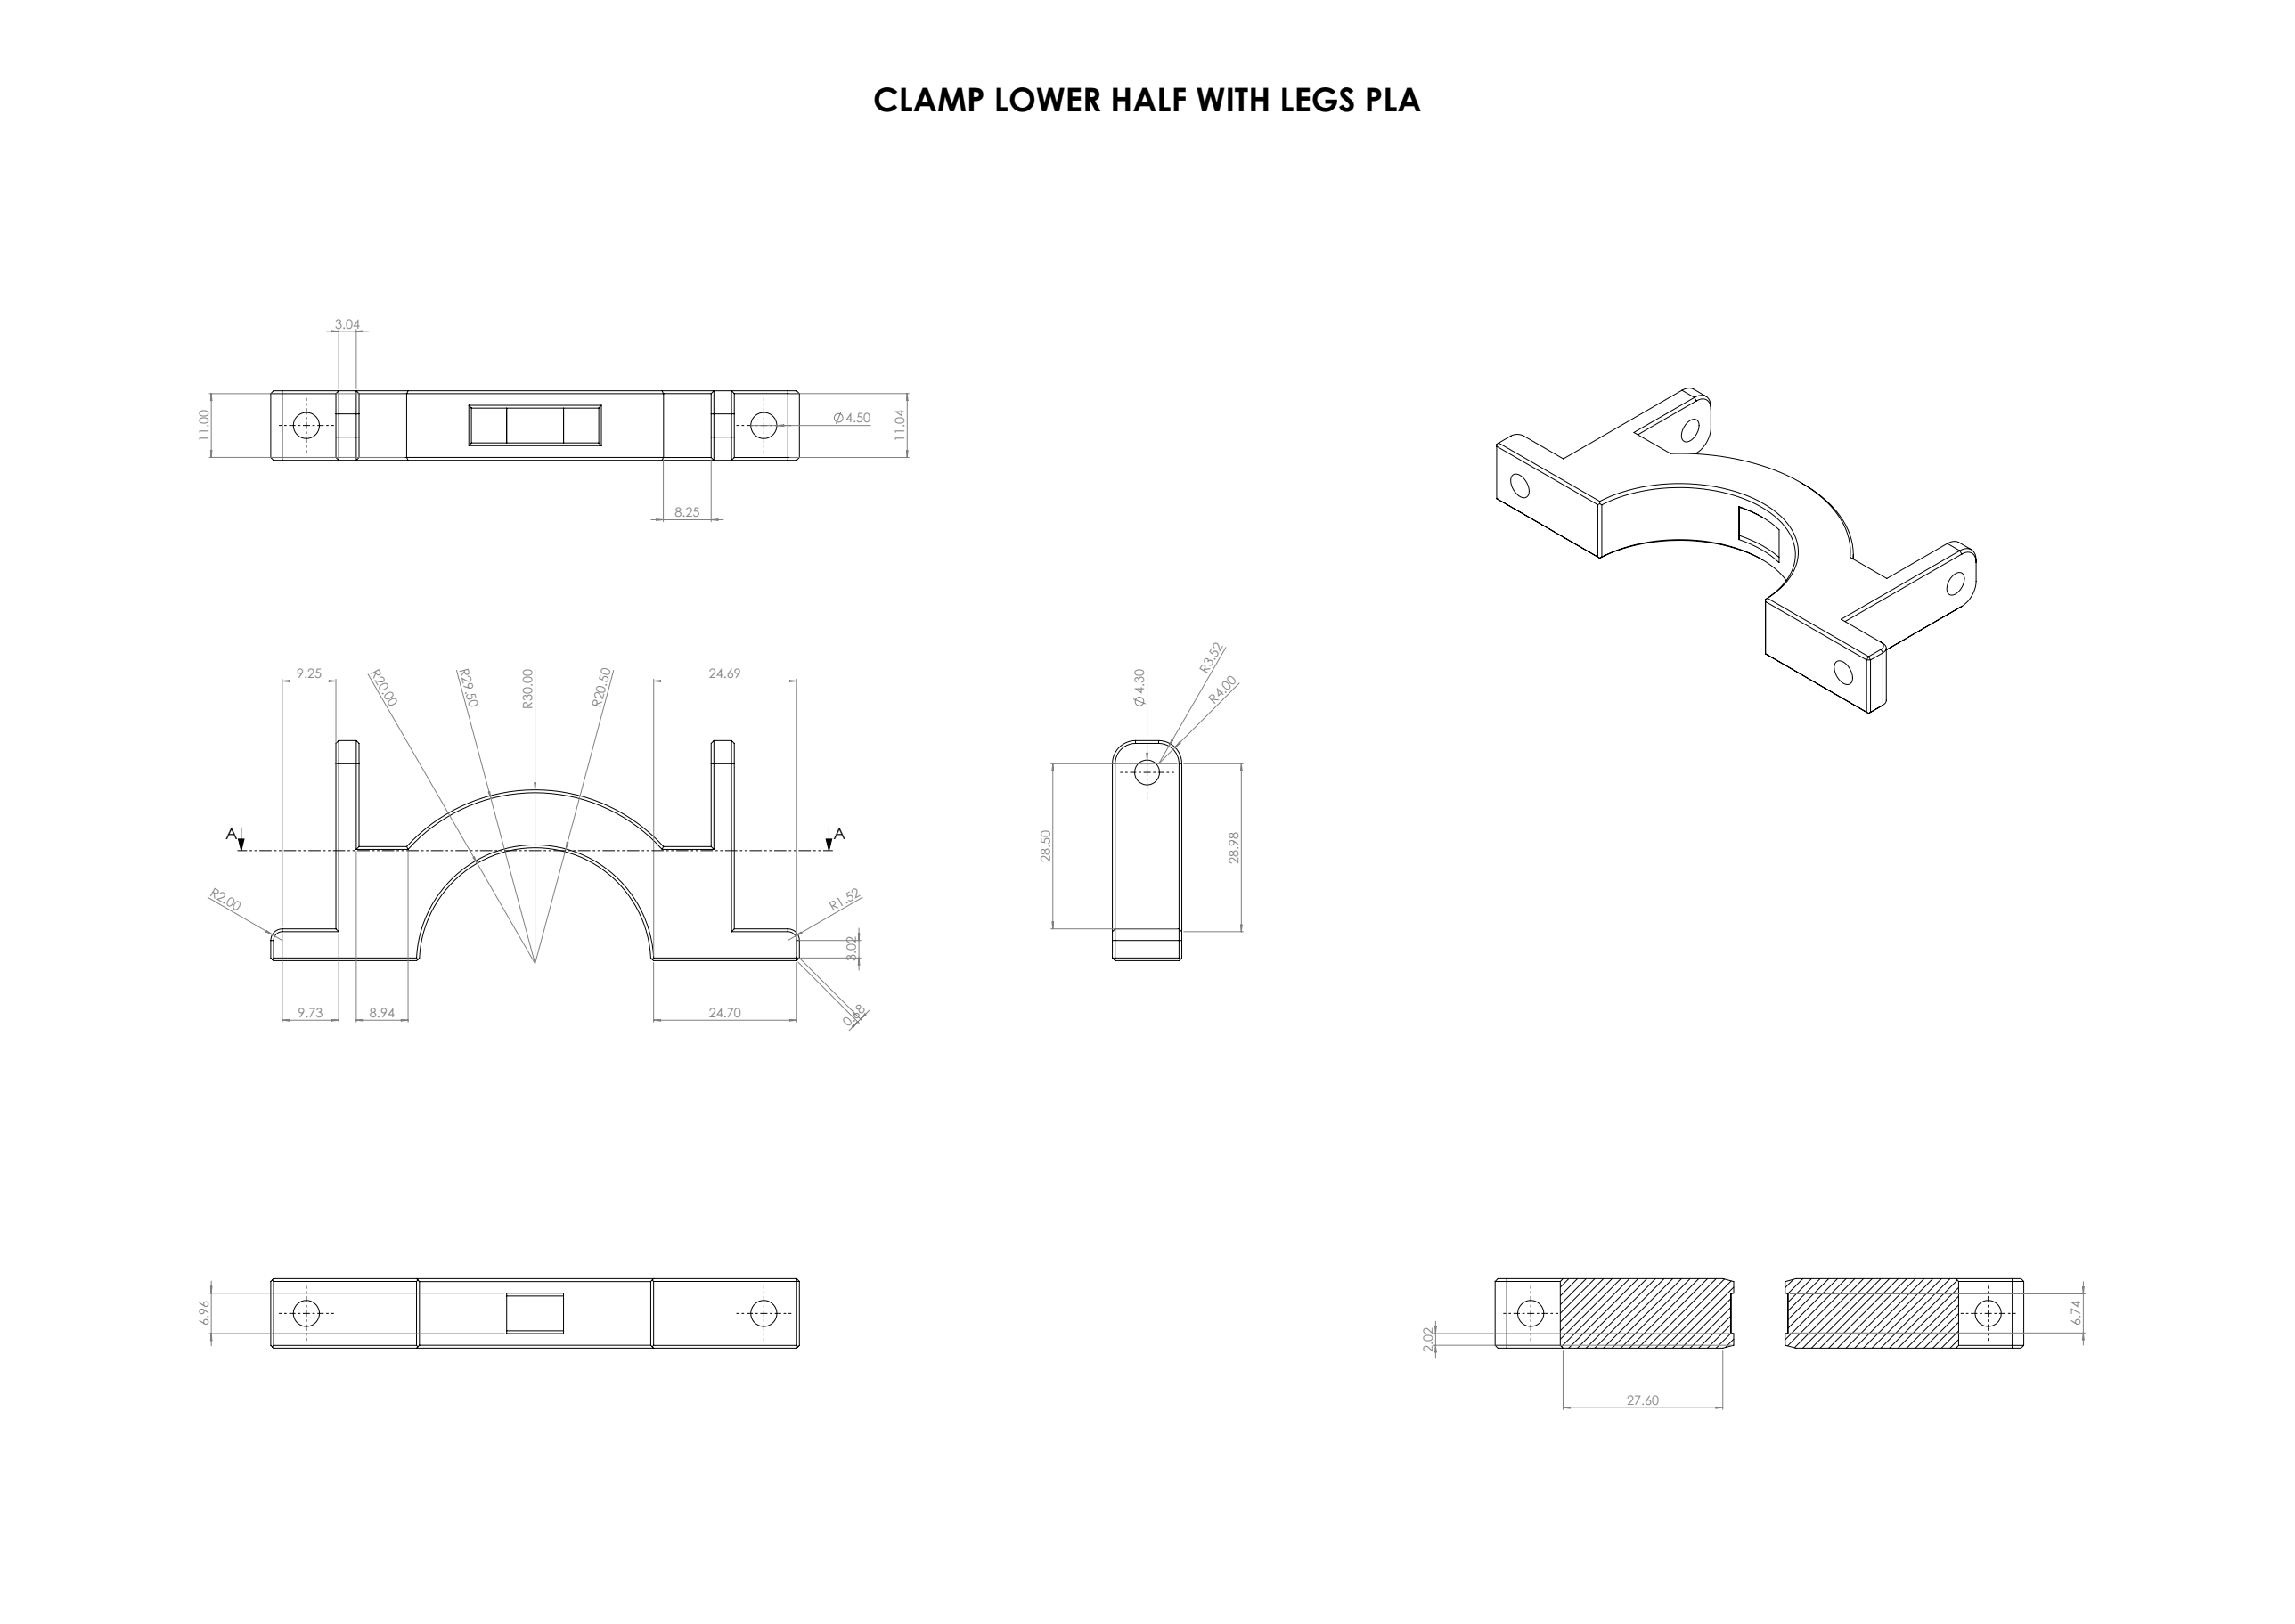
ISO-10303-21;
HEADER;
/* Generated by software containing ST-Developer
 * from STEP Tools, Inc. (www.steptools.com) 
 */

FILE_DESCRIPTION(
/* description */ (''),
/* implementation_level */ '2;1');

FILE_NAME(
/* name */ '02_Clamp_Lower_Half_with_Legs_PLA.step',
/* time_stamp */ '2026-10-21T02:01:14-07:00',
/* author */ (''),
/* organization */ (''),
/* preprocessor_version */ 'ST-DEVELOPER v20.2',
/* originating_system */ 'Autodesk Translation Framework v15.15.0.0',
/* authorisation */ '');

FILE_SCHEMA (('AUTOMOTIVE_DESIGN { 1 0 10303 214 3 1 1 }'));
ENDSEC;

DATA;
#10=MECHANICAL_DESIGN_GEOMETRIC_PRESENTATION_REPRESENTATION('',(#615),#37181);
#120=B_SPLINE_CURVE_WITH_KNOTS('',3,(#20379,#20380,#20381,#20382),
 .UNSPECIFIED.,.F.,.F.,(4,4),(-0.0159210516924088,0.),.UNSPECIFIED.);
#121=B_SPLINE_CURVE_WITH_KNOTS('',3,(#20385,#20386,#20387,#20388),
 .UNSPECIFIED.,.F.,.F.,(4,4),(-0.0159210527656447,0.),.UNSPECIFIED.);
#122=B_SPLINE_CURVE_WITH_KNOTS('',3,(#20391,#20392,#20393,#20394),
 .UNSPECIFIED.,.F.,.F.,(4,4),(-0.0159210517190927,0.),.UNSPECIFIED.);
#123=B_SPLINE_CURVE_WITH_KNOTS('',3,(#20397,#20398,#20399,#20400),
 .UNSPECIFIED.,.F.,.F.,(4,4),(-0.0159210527692958,0.),.UNSPECIFIED.);
#124=B_SPLINE_CURVE_WITH_KNOTS('',3,(#20440,#20441,#20442,#20443),
 .UNSPECIFIED.,.F.,.F.,(4,4),(-0.0698067370947057,0.),.UNSPECIFIED.);
#125=B_SPLINE_CURVE_WITH_KNOTS('',3,(#20446,#20447,#20448,#20449),
 .UNSPECIFIED.,.F.,.F.,(4,4),(-0.0698065886608642,0.),.UNSPECIFIED.);
#126=B_SPLINE_CURVE_WITH_KNOTS('',3,(#20455,#20456,#20457,#20458),
 .UNSPECIFIED.,.F.,.F.,(4,4),(-0.0698067370949415,0.),.UNSPECIFIED.);
#127=B_SPLINE_CURVE_WITH_KNOTS('',3,(#20461,#20462,#20463,#20464),
 .UNSPECIFIED.,.F.,.F.,(4,4),(-0.0698065886603473,0.),.UNSPECIFIED.);
#589=SHAPE_REPRESENTATION_RELATIONSHIP('SRR','None',#37239,#602);
#602=ADVANCED_BREP_SHAPE_REPRESENTATION('',(#628),#37169);
#615=STYLED_ITEM('',(#37387),#628);
#628=MANIFOLD_SOLID_BREP('Body1',#14777);
#644=FACE_BOUND('',#2261,.T.);
#645=FACE_BOUND('',#2293,.T.);
#646=FACE_BOUND('',#2303,.T.);
#647=FACE_BOUND('',#2305,.T.);
#648=FACE_BOUND('',#2313,.T.);
#649=FACE_BOUND('',#2321,.T.);
#650=FACE_BOUND('',#2336,.T.);
#651=FACE_BOUND('',#2339,.T.);
#652=FACE_BOUND('',#2351,.T.);
#653=FACE_BOUND('',#2354,.T.);
#696=CYLINDRICAL_SURFACE('',#15034,4.);
#697=CYLINDRICAL_SURFACE('',#15036,4.);
#698=CYLINDRICAL_SURFACE('',#15051,2.);
#699=CYLINDRICAL_SURFACE('',#15094,20.);
#700=CYLINDRICAL_SURFACE('',#15116,30.);
#701=CYLINDRICAL_SURFACE('',#15125,2.25);
#702=CYLINDRICAL_SURFACE('',#15126,2.25);
#703=CYLINDRICAL_SURFACE('',#15128,2.15);
#704=CYLINDRICAL_SURFACE('',#15130,2.15);
#705=CYLINDRICAL_SURFACE('',#15131,4.);
#706=CYLINDRICAL_SURFACE('',#15132,4.);
#707=CYLINDRICAL_SURFACE('',#15133,2.);
#971=CIRCLE('',#15000,4.);
#972=CIRCLE('',#15001,3.52);
#973=CIRCLE('',#15004,4.);
#974=CIRCLE('',#15005,3.52);
#975=CIRCLE('',#15009,2.15);
#976=CIRCLE('',#15015,2.);
#977=CIRCLE('',#15016,1.52);
#978=CIRCLE('',#15019,4.);
#979=CIRCLE('',#15020,3.52);
#980=CIRCLE('',#15023,4.);
#981=CIRCLE('',#15024,3.52);
#982=CIRCLE('',#15027,2.);
#983=CIRCLE('',#15028,1.52);
#984=CIRCLE('',#15031,29.5);
#985=CIRCLE('',#15032,1.52);
#986=CIRCLE('',#15033,20.5);
#987=CIRCLE('',#15038,20.5);
#988=CIRCLE('',#15039,1.52);
#989=CIRCLE('',#15040,29.5);
#990=CIRCLE('',#15048,2.);
#991=CIRCLE('',#15052,2.);
#992=CIRCLE('',#15057,2.25);
#993=CIRCLE('',#15063,4.);
#994=CIRCLE('',#15064,3.52);
#995=CIRCLE('',#15067,4.);
#996=CIRCLE('',#15068,3.52);
#997=CIRCLE('',#15071,2.25);
#998=CIRCLE('',#15073,2.15);
#999=CIRCLE('',#15077,4.);
#1000=CIRCLE('',#15078,3.52);
#1001=CIRCLE('',#15081,4.);
#1002=CIRCLE('',#15082,3.52);
#1003=CIRCLE('',#15085,2.15);
#1004=CIRCLE('',#15090,20.);
#1005=CIRCLE('',#15093,20.);
#1006=CIRCLE('',#15095,20.);
#1007=CIRCLE('',#15096,20.);
#1008=CIRCLE('',#15101,20.48);
#1009=CIRCLE('',#15103,20.48);
#1010=CIRCLE('',#15105,29.52);
#1011=CIRCLE('',#15110,30.);
#1012=CIRCLE('',#15112,30.);
#1013=CIRCLE('',#15113,29.52);
#1014=CIRCLE('',#15117,30.);
#1015=CIRCLE('',#15118,30.);
#1016=CIRCLE('',#15121,2.25);
#1017=CIRCLE('',#15127,2.25);
#1018=CIRCLE('',#15129,2.15);
#1291=CONICAL_SURFACE('',#14999,3.76,0.785398163397446);
#1292=CONICAL_SURFACE('',#15003,3.76,0.785398163397446);
#1293=CONICAL_SURFACE('',#15014,1.76,0.78539816339745);
#1294=CONICAL_SURFACE('',#15018,3.76,0.785398163397446);
#1295=CONICAL_SURFACE('',#15022,3.76,0.785398163397446);
#1296=CONICAL_SURFACE('',#15026,1.76,0.78539816339745);
#1297=CONICAL_SURFACE('',#15047,1.76,0.785398163397452);
#1298=CONICAL_SURFACE('',#15059,1.76,0.785398163397452);
#1299=CONICAL_SURFACE('',#15062,3.76,0.785398163397446);
#1300=CONICAL_SURFACE('',#15066,3.76,0.785398163397446);
#1301=CONICAL_SURFACE('',#15076,3.76,0.785398163397446);
#1302=CONICAL_SURFACE('',#15080,3.76,0.785398163397446);
#1303=CONICAL_SURFACE('',#15089,20.25,0.785398163397446);
#1304=CONICAL_SURFACE('',#15092,20.25,0.785398163397446);
#1305=CONICAL_SURFACE('',#15100,20.24,0.785398163397448);
#1306=CONICAL_SURFACE('',#15102,20.24,0.785398163397449);
#1307=CONICAL_SURFACE('',#15109,29.76,0.785398163397449);
#1308=CONICAL_SURFACE('',#15111,29.76,0.785398163397448);
#1309=CONICAL_SURFACE('',#15119,29.75,0.785398163397446);
#1310=CONICAL_SURFACE('',#15122,29.75,0.785398163397446);
#1410=FACE_OUTER_BOUND('',#2254,.T.);
#1411=FACE_OUTER_BOUND('',#2255,.T.);
#1412=FACE_OUTER_BOUND('',#2256,.T.);
#1413=FACE_OUTER_BOUND('',#2257,.T.);
#1414=FACE_OUTER_BOUND('',#2258,.T.);
#1415=FACE_OUTER_BOUND('',#2259,.T.);
#1416=FACE_OUTER_BOUND('',#2260,.T.);
#1417=FACE_OUTER_BOUND('',#2262,.T.);
#1418=FACE_OUTER_BOUND('',#2263,.T.);
#1419=FACE_OUTER_BOUND('',#2264,.T.);
#1420=FACE_OUTER_BOUND('',#2265,.T.);
#1421=FACE_OUTER_BOUND('',#2266,.T.);
#1422=FACE_OUTER_BOUND('',#2267,.T.);
#1423=FACE_OUTER_BOUND('',#2268,.T.);
#1424=FACE_OUTER_BOUND('',#2269,.T.);
#1425=FACE_OUTER_BOUND('',#2270,.T.);
#1426=FACE_OUTER_BOUND('',#2271,.T.);
#1427=FACE_OUTER_BOUND('',#2272,.T.);
#1428=FACE_OUTER_BOUND('',#2273,.T.);
#1429=FACE_OUTER_BOUND('',#2274,.T.);
#1430=FACE_OUTER_BOUND('',#2275,.T.);
#1431=FACE_OUTER_BOUND('',#2276,.T.);
#1432=FACE_OUTER_BOUND('',#2277,.T.);
#1433=FACE_OUTER_BOUND('',#2278,.T.);
#1434=FACE_OUTER_BOUND('',#2279,.T.);
#1435=FACE_OUTER_BOUND('',#2280,.T.);
#1436=FACE_OUTER_BOUND('',#2281,.T.);
#1437=FACE_OUTER_BOUND('',#2282,.T.);
#1438=FACE_OUTER_BOUND('',#2283,.T.);
#1439=FACE_OUTER_BOUND('',#2284,.T.);
#1440=FACE_OUTER_BOUND('',#2285,.T.);
#1441=FACE_OUTER_BOUND('',#2286,.T.);
#1442=FACE_OUTER_BOUND('',#2287,.T.);
#1443=FACE_OUTER_BOUND('',#2288,.T.);
#1444=FACE_OUTER_BOUND('',#2289,.T.);
#1445=FACE_OUTER_BOUND('',#2290,.T.);
#1446=FACE_OUTER_BOUND('',#2291,.T.);
#1447=FACE_OUTER_BOUND('',#2292,.T.);
#1448=FACE_OUTER_BOUND('',#2294,.T.);
#1449=FACE_OUTER_BOUND('',#2295,.T.);
#1450=FACE_OUTER_BOUND('',#2296,.T.);
#1451=FACE_OUTER_BOUND('',#2297,.T.);
#1452=FACE_OUTER_BOUND('',#2298,.T.);
#1453=FACE_OUTER_BOUND('',#2299,.T.);
#1454=FACE_OUTER_BOUND('',#2300,.T.);
#1455=FACE_OUTER_BOUND('',#2301,.T.);
#1456=FACE_OUTER_BOUND('',#2302,.T.);
#1457=FACE_OUTER_BOUND('',#2304,.T.);
#1458=FACE_OUTER_BOUND('',#2306,.T.);
#1459=FACE_OUTER_BOUND('',#2307,.T.);
#1460=FACE_OUTER_BOUND('',#2308,.T.);
#1461=FACE_OUTER_BOUND('',#2309,.T.);
#1462=FACE_OUTER_BOUND('',#2310,.T.);
#1463=FACE_OUTER_BOUND('',#2311,.T.);
#1464=FACE_OUTER_BOUND('',#2312,.T.);
#1465=FACE_OUTER_BOUND('',#2314,.T.);
#1466=FACE_OUTER_BOUND('',#2315,.T.);
#1467=FACE_OUTER_BOUND('',#2316,.T.);
#1468=FACE_OUTER_BOUND('',#2317,.T.);
#1469=FACE_OUTER_BOUND('',#2318,.T.);
#1470=FACE_OUTER_BOUND('',#2319,.T.);
#1471=FACE_OUTER_BOUND('',#2320,.T.);
#1472=FACE_OUTER_BOUND('',#2322,.T.);
#1473=FACE_OUTER_BOUND('',#2323,.T.);
#1474=FACE_OUTER_BOUND('',#2324,.T.);
#1475=FACE_OUTER_BOUND('',#2325,.T.);
#1476=FACE_OUTER_BOUND('',#2326,.T.);
#1477=FACE_OUTER_BOUND('',#2327,.T.);
#1478=FACE_OUTER_BOUND('',#2328,.T.);
#1479=FACE_OUTER_BOUND('',#2329,.T.);
#1480=FACE_OUTER_BOUND('',#2330,.T.);
#1481=FACE_OUTER_BOUND('',#2331,.T.);
#1482=FACE_OUTER_BOUND('',#2332,.T.);
#1483=FACE_OUTER_BOUND('',#2333,.T.);
#1484=FACE_OUTER_BOUND('',#2334,.T.);
#1485=FACE_OUTER_BOUND('',#2335,.T.);
#1486=FACE_OUTER_BOUND('',#2337,.T.);
#1487=FACE_OUTER_BOUND('',#2338,.T.);
#1488=FACE_OUTER_BOUND('',#2340,.T.);
#1489=FACE_OUTER_BOUND('',#2341,.T.);
#1490=FACE_OUTER_BOUND('',#2342,.T.);
#1491=FACE_OUTER_BOUND('',#2343,.T.);
#1492=FACE_OUTER_BOUND('',#2344,.T.);
#1493=FACE_OUTER_BOUND('',#2345,.T.);
#1494=FACE_OUTER_BOUND('',#2346,.T.);
#1495=FACE_OUTER_BOUND('',#2347,.T.);
#1496=FACE_OUTER_BOUND('',#2348,.T.);
#1497=FACE_OUTER_BOUND('',#2349,.T.);
#1498=FACE_OUTER_BOUND('',#2350,.T.);
#1499=FACE_OUTER_BOUND('',#2352,.T.);
#1500=FACE_OUTER_BOUND('',#2353,.T.);
#2254=EDGE_LOOP('',(#9371,#9372,#9373,#9374));
#2255=EDGE_LOOP('',(#9375,#9376,#9377,#9378));
#2256=EDGE_LOOP('',(#9379,#9380,#9381,#9382));
#2257=EDGE_LOOP('',(#9383,#9384,#9385,#9386));
#2258=EDGE_LOOP('',(#9387,#9388,#9389,#9390));
#2259=EDGE_LOOP('',(#9391,#9392,#9393,#9394));
#2260=EDGE_LOOP('',(#9395,#9396,#9397,#9398,#9399,#9400));
#2261=EDGE_LOOP('',(#9401));
#2262=EDGE_LOOP('',(#9402,#9403,#9404,#9405,#9406,#9407));
#2263=EDGE_LOOP('',(#9408,#9409,#9410,#9411));
#2264=EDGE_LOOP('',(#9412,#9413,#9414,#9415));
#2265=EDGE_LOOP('',(#9416,#9417,#9418,#9419));
#2266=EDGE_LOOP('',(#9420,#9421,#9422,#9423));
#2267=EDGE_LOOP('',(#9424,#9425,#9426,#9427,#9428));
#2268=EDGE_LOOP('',(#9429,#9430,#9431,#9432));
#2269=EDGE_LOOP('',(#9433,#9434,#9435,#9436));
#2270=EDGE_LOOP('',(#9437,#9438,#9439,#9440));
#2271=EDGE_LOOP('',(#9441,#9442,#9443,#9444));
#2272=EDGE_LOOP('',(#9445,#9446,#9447,#9448));
#2273=EDGE_LOOP('',(#9449,#9450,#9451,#9452,#9453));
#2274=EDGE_LOOP('',(#9454,#9455,#9456,#9457,#9458,#9459,#9460,#9461,#9462,
#9463,#9464,#9465,#9466,#9467,#9468,#9469,#9470,#9471));
#2275=EDGE_LOOP('',(#9472,#9473,#9474,#9475));
#2276=EDGE_LOOP('',(#9476,#9477,#9478,#9479));
#2277=EDGE_LOOP('',(#9480,#9481,#9482,#9483));
#2278=EDGE_LOOP('',(#9484,#9485,#9486,#9487,#9488,#9489,#9490,#9491,#9492,
#9493,#9494,#9495,#9496,#9497,#9498,#9499,#9500,#9501));
#2279=EDGE_LOOP('',(#9502,#9503,#9504,#9505,#9506,#9507));
#2280=EDGE_LOOP('',(#9508,#9509,#9510,#9511));
#2281=EDGE_LOOP('',(#9512,#9513,#9514,#9515,#9516,#9517));
#2282=EDGE_LOOP('',(#9518,#9519,#9520));
#2283=EDGE_LOOP('',(#9521,#9522,#9523,#9524,#9525));
#2284=EDGE_LOOP('',(#9526,#9527,#9528,#9529));
#2285=EDGE_LOOP('',(#9530,#9531,#9532,#9533));
#2286=EDGE_LOOP('',(#9534,#9535,#9536,#9537));
#2287=EDGE_LOOP('',(#9538,#9539,#9540,#9541,#9542));
#2288=EDGE_LOOP('',(#9543,#9544,#9545,#9546));
#2289=EDGE_LOOP('',(#9547,#9548,#9549,#9550));
#2290=EDGE_LOOP('',(#9551,#9552,#9553,#9554,#9555));
#2291=EDGE_LOOP('',(#9556,#9557,#9558,#9559,#9560,#9561));
#2292=EDGE_LOOP('',(#9562,#9563,#9564,#9565));
#2293=EDGE_LOOP('',(#9566));
#2294=EDGE_LOOP('',(#9567,#9568,#9569,#9570,#9571,#9572));
#2295=EDGE_LOOP('',(#9573,#9574,#9575,#9576));
#2296=EDGE_LOOP('',(#9577,#9578,#9579,#9580));
#2297=EDGE_LOOP('',(#9581,#9582,#9583,#9584));
#2298=EDGE_LOOP('',(#9585,#9586,#9587,#9588));
#2299=EDGE_LOOP('',(#9589,#9590,#9591,#9592));
#2300=EDGE_LOOP('',(#9593,#9594,#9595,#9596));
#2301=EDGE_LOOP('',(#9597,#9598,#9599,#9600));
#2302=EDGE_LOOP('',(#9601,#9602,#9603,#9604));
#2303=EDGE_LOOP('',(#9605));
#2304=EDGE_LOOP('',(#9606,#9607,#9608,#9609,#9610,#9611));
#2305=EDGE_LOOP('',(#9612));
#2306=EDGE_LOOP('',(#9613,#9614,#9615,#9616));
#2307=EDGE_LOOP('',(#9617,#9618,#9619,#9620));
#2308=EDGE_LOOP('',(#9621,#9622,#9623,#9624));
#2309=EDGE_LOOP('',(#9625,#9626,#9627,#9628));
#2310=EDGE_LOOP('',(#9629,#9630,#9631,#9632));
#2311=EDGE_LOOP('',(#9633,#9634,#9635,#9636));
#2312=EDGE_LOOP('',(#9637,#9638,#9639,#9640,#9641,#9642));
#2313=EDGE_LOOP('',(#9643));
#2314=EDGE_LOOP('',(#9644,#9645,#9646,#9647));
#2315=EDGE_LOOP('',(#9648,#9649,#9650,#9651,#9652,#9653));
#2316=EDGE_LOOP('',(#9654,#9655,#9656,#9657,#9658,#9659));
#2317=EDGE_LOOP('',(#9660,#9661,#9662,#9663,#9664,#9665));
#2318=EDGE_LOOP('',(#9666,#9667,#9668,#9669));
#2319=EDGE_LOOP('',(#9670,#9671,#9672,#9673,#9674,#9675));
#2320=EDGE_LOOP('',(#9676,#9677,#9678,#9679));
#2321=EDGE_LOOP('',(#9680,#9681,#9682,#9683));
#2322=EDGE_LOOP('',(#9684,#9685,#9686,#9687,#9688,#9689));
#2323=EDGE_LOOP('',(#9690,#9691,#9692,#9693));
#2324=EDGE_LOOP('',(#9694,#9695,#9696,#9697));
#2325=EDGE_LOOP('',(#9698,#9699,#9700,#9701,#9702,#9703));
#2326=EDGE_LOOP('',(#9704,#9705,#9706,#9707,#9708,#9709));
#2327=EDGE_LOOP('',(#9710,#9711,#9712,#9713,#9714,#9715));
#2328=EDGE_LOOP('',(#9716,#9717,#9718,#9719,#9720,#9721));
#2329=EDGE_LOOP('',(#9722,#9723,#9724,#9725));
#2330=EDGE_LOOP('',(#9726,#9727,#9728,#9729));
#2331=EDGE_LOOP('',(#9730,#9731,#9732,#9733,#9734,#9735));
#2332=EDGE_LOOP('',(#9736,#9737,#9738,#9739,#9740,#9741));
#2333=EDGE_LOOP('',(#9742,#9743,#9744,#9745,#9746,#9747));
#2334=EDGE_LOOP('',(#9748,#9749,#9750,#9751,#9752,#9753));
#2335=EDGE_LOOP('',(#9754,#9755,#9756,#9757));
#2336=EDGE_LOOP('',(#9758,#9759,#9760,#9761));
#2337=EDGE_LOOP('',(#9762,#9763,#9764,#9765,#9766,#9767));
#2338=EDGE_LOOP('',(#9768,#9769,#9770,#9771));
#2339=EDGE_LOOP('',(#9772));
#2340=EDGE_LOOP('',(#9773,#9774,#9775,#9776,#9777,#9778));
#2341=EDGE_LOOP('',(#9779,#9780,#9781,#9782,#9783,#9784));
#2342=EDGE_LOOP('',(#9785,#9786,#9787,#9788,#9789,#9790));
#2343=EDGE_LOOP('',(#9791,#9792,#9793,#9794));
#2344=EDGE_LOOP('',(#9795,#9796,#9797,#9798));
#2345=EDGE_LOOP('',(#9799,#9800,#9801,#9802));
#2346=EDGE_LOOP('',(#9803,#9804,#9805,#9806));
#2347=EDGE_LOOP('',(#9807,#9808,#9809,#9810));
#2348=EDGE_LOOP('',(#9811,#9812,#9813,#9814));
#2349=EDGE_LOOP('',(#9815,#9816,#9817,#9818));
#2350=EDGE_LOOP('',(#9819,#9820,#9821,#9822));
#2351=EDGE_LOOP('',(#9823));
#2352=EDGE_LOOP('',(#9824,#9825,#9826,#9827));
#2353=EDGE_LOOP('',(#9828,#9829,#9830,#9831,#9832,#9833));
#2354=EDGE_LOOP('',(#9834));
#3114=(
BOUNDED_CURVE()
B_SPLINE_CURVE(2,(#20022,#20023,#20024),.UNSPECIFIED.,.F.,.F.)
B_SPLINE_CURVE_WITH_KNOTS((3,3),(0.,0.0711434865298028),.UNSPECIFIED.)
CURVE()
GEOMETRIC_REPRESENTATION_ITEM()
RATIONAL_B_SPLINE_CURVE((1.,1.,1.))
REPRESENTATION_ITEM('')
);
#3115=(
BOUNDED_CURVE()
B_SPLINE_CURVE(2,(#20032,#20033,#20034),.UNSPECIFIED.,.F.,.F.)
B_SPLINE_CURVE_WITH_KNOTS((3,3),(0.0811630519003425,0.084492689542221),
 .UNSPECIFIED.)
CURVE()
GEOMETRIC_REPRESENTATION_ITEM()
RATIONAL_B_SPLINE_CURVE((1.0000049607761,1.00000258214363,1.))
REPRESENTATION_ITEM('')
);
#3116=(
BOUNDED_CURVE()
B_SPLINE_CURVE(2,(#20038,#20039,#20040),.UNSPECIFIED.,.F.,.F.)
B_SPLINE_CURVE_WITH_KNOTS((3,3),(0.,0.00332963764187841),.UNSPECIFIED.)
CURVE()
GEOMETRIC_REPRESENTATION_ITEM()
RATIONAL_B_SPLINE_CURVE((1.,1.00000258214363,1.0000049607761))
REPRESENTATION_ITEM('')
);
#3117=(
BOUNDED_CURVE()
B_SPLINE_CURVE(2,(#20175,#20176,#20177),.UNSPECIFIED.,.F.,.F.)
B_SPLINE_CURVE_WITH_KNOTS((3,3),(0.0429017134859085,0.0855944597309053),
 .UNSPECIFIED.)
CURVE()
GEOMETRIC_REPRESENTATION_ITEM()
RATIONAL_B_SPLINE_CURVE((1.,1.,1.))
REPRESENTATION_ITEM('')
);
#3118=(
BOUNDED_CURVE()
B_SPLINE_CURVE(2,(#20183,#20184,#20185),.UNSPECIFIED.,.F.,.F.)
B_SPLINE_CURVE_WITH_KNOTS((3,3),(0.,0.0711434865298028),.UNSPECIFIED.)
CURVE()
GEOMETRIC_REPRESENTATION_ITEM()
RATIONAL_B_SPLINE_CURVE((1.,1.,1.))
REPRESENTATION_ITEM('')
);
#3119=(
BOUNDED_CURVE()
B_SPLINE_CURVE(2,(#20192,#20193,#20194),.UNSPECIFIED.,.F.,.F.)
B_SPLINE_CURVE_WITH_KNOTS((3,3),(0.081163051900335,0.0844926895422209),
 .UNSPECIFIED.)
CURVE()
GEOMETRIC_REPRESENTATION_ITEM()
RATIONAL_B_SPLINE_CURVE((1.00000496077593,1.00000258214354,1.))
REPRESENTATION_ITEM('')
);
#3120=(
BOUNDED_CURVE()
B_SPLINE_CURVE(2,(#20197,#20198,#20199),.UNSPECIFIED.,.F.,.F.)
B_SPLINE_CURVE_WITH_KNOTS((3,3),(0.,0.00332963764188661),.UNSPECIFIED.)
CURVE()
GEOMETRIC_REPRESENTATION_ITEM()
RATIONAL_B_SPLINE_CURVE((1.,1.00000258214354,1.00000496077593))
REPRESENTATION_ITEM('')
);
#3121=(
BOUNDED_CURVE()
B_SPLINE_CURVE(2,(#20231,#20232,#20233),.UNSPECIFIED.,.F.,.F.)
B_SPLINE_CURVE_WITH_KNOTS((3,3),(0.,0.0426927462449967),.UNSPECIFIED.)
CURVE()
GEOMETRIC_REPRESENTATION_ITEM()
RATIONAL_B_SPLINE_CURVE((1.,1.,1.))
REPRESENTATION_ITEM('')
);
#3122=(
BOUNDED_CURVE()
B_SPLINE_CURVE(2,(#20250,#20251,#20252),.UNSPECIFIED.,.F.,.F.)
B_SPLINE_CURVE_WITH_KNOTS((3,3),(0.0429017134858602,0.0855944597309048),
 .UNSPECIFIED.)
CURVE()
GEOMETRIC_REPRESENTATION_ITEM()
RATIONAL_B_SPLINE_CURVE((1.,1.,1.))
REPRESENTATION_ITEM('')
);
#3123=(
BOUNDED_CURVE()
B_SPLINE_CURVE(2,(#20259,#20260,#20261),.UNSPECIFIED.,.F.,.F.)
B_SPLINE_CURVE_WITH_KNOTS((3,3),(0.043419103644769,0.0876516150043356),
 .UNSPECIFIED.)
CURVE()
GEOMETRIC_REPRESENTATION_ITEM()
RATIONAL_B_SPLINE_CURVE((1.00007900493187,1.00007974496581,1.))
REPRESENTATION_ITEM('')
);
#3124=(
BOUNDED_CURVE()
B_SPLINE_CURVE(2,(#20264,#20265,#20266),.UNSPECIFIED.,.F.,.F.)
B_SPLINE_CURVE_WITH_KNOTS((3,3),(0.,0.044232511359626),.UNSPECIFIED.)
CURVE()
GEOMETRIC_REPRESENTATION_ITEM()
RATIONAL_B_SPLINE_CURVE((1.,1.00007974496639,1.00007900493244))
REPRESENTATION_ITEM('')
);
#3125=(
BOUNDED_CURVE()
B_SPLINE_CURVE(2,(#20309,#20310,#20311),.UNSPECIFIED.,.F.,.F.)
B_SPLINE_CURVE_WITH_KNOTS((3,3),(0.,0.0711434865298029),.UNSPECIFIED.)
CURVE()
GEOMETRIC_REPRESENTATION_ITEM()
RATIONAL_B_SPLINE_CURVE((1.,1.,1.))
REPRESENTATION_ITEM('')
);
#3126=(
BOUNDED_CURVE()
B_SPLINE_CURVE(2,(#20335,#20336,#20337),.UNSPECIFIED.,.F.,.F.)
B_SPLINE_CURVE_WITH_KNOTS((3,3),(0.,0.0711434865298029),.UNSPECIFIED.)
CURVE()
GEOMETRIC_REPRESENTATION_ITEM()
RATIONAL_B_SPLINE_CURVE((1.,1.,1.))
REPRESENTATION_ITEM('')
);
#3127=(
BOUNDED_CURVE()
B_SPLINE_CURVE(2,(#20340,#20341,#20342),.UNSPECIFIED.,.F.,.F.)
B_SPLINE_CURVE_WITH_KNOTS((3,3),(0.,0.0426927462450447),.UNSPECIFIED.)
CURVE()
GEOMETRIC_REPRESENTATION_ITEM()
RATIONAL_B_SPLINE_CURVE((1.,1.,1.))
REPRESENTATION_ITEM('')
);
#3128=(
BOUNDED_CURVE()
B_SPLINE_CURVE(2,(#20354,#20355,#20356),.UNSPECIFIED.,.F.,.F.)
B_SPLINE_CURVE_WITH_KNOTS((3,3),(0.0434191036447888,0.0876516150043351),
 .UNSPECIFIED.)
CURVE()
GEOMETRIC_REPRESENTATION_ITEM()
RATIONAL_B_SPLINE_CURVE((1.00007900493244,1.00007974496639,1.))
REPRESENTATION_ITEM('')
);
#3129=(
BOUNDED_CURVE()
B_SPLINE_CURVE(2,(#20361,#20362,#20363),.UNSPECIFIED.,.F.,.F.)
B_SPLINE_CURVE_WITH_KNOTS((3,3),(0.,0.0442325113596284),.UNSPECIFIED.)
CURVE()
GEOMETRIC_REPRESENTATION_ITEM()
RATIONAL_B_SPLINE_CURVE((1.,1.00007974496678,1.00007900493282))
REPRESENTATION_ITEM('')
);
#3130=(
BOUNDED_CURVE()
B_SPLINE_CURVE(2,(#20405,#20406,#20407),.UNSPECIFIED.,.F.,.F.)
B_SPLINE_CURVE_WITH_KNOTS((3,3),(-3.26709460117384,-3.09375460254933),
 .UNSPECIFIED.)
CURVE()
GEOMETRIC_REPRESENTATION_ITEM()
RATIONAL_B_SPLINE_CURVE((1.22511255627814,1.2314549978879,1.23649074068738))
REPRESENTATION_ITEM('')
);
#3131=(
BOUNDED_CURVE()
B_SPLINE_CURVE(2,(#20408,#20409,#20410),.UNSPECIFIED.,.F.,.F.)
B_SPLINE_CURVE_WITH_KNOTS((3,3),(-1.75772269823236,-1.58438269960785),
 .UNSPECIFIED.)
CURVE()
GEOMETRIC_REPRESENTATION_ITEM()
RATIONAL_B_SPLINE_CURVE((1.23649074068738,1.2314549978879,1.22511255627814))
REPRESENTATION_ITEM('')
);
#3132=(
BOUNDED_CURVE()
B_SPLINE_CURVE(2,(#20413,#20414,#20415),.UNSPECIFIED.,.F.,.F.)
B_SPLINE_CURVE_WITH_KNOTS((3,3),(-1.75772269823236,-1.58438269960785),
 .UNSPECIFIED.)
CURVE()
GEOMETRIC_REPRESENTATION_ITEM()
RATIONAL_B_SPLINE_CURVE((1.23649074068738,1.2314549978879,1.22511255627814))
REPRESENTATION_ITEM('')
);
#3133=(
BOUNDED_CURVE()
B_SPLINE_CURVE(2,(#20418,#20419,#20420),.UNSPECIFIED.,.F.,.F.)
B_SPLINE_CURVE_WITH_KNOTS((3,3),(-3.26709460117384,-3.09375460254933),
 .UNSPECIFIED.)
CURVE()
GEOMETRIC_REPRESENTATION_ITEM()
RATIONAL_B_SPLINE_CURVE((1.22511255627814,1.2314549978879,1.23649074068738))
REPRESENTATION_ITEM('')
);
#3134=(
BOUNDED_CURVE()
B_SPLINE_CURVE(2,(#20466,#20467,#20468),.UNSPECIFIED.,.F.,.F.)
B_SPLINE_CURVE_WITH_KNOTS((3,3),(-0.360391606906832,-0.356059784727892),
 .UNSPECIFIED.)
CURVE()
GEOMETRIC_REPRESENTATION_ITEM()
RATIONAL_B_SPLINE_CURVE((1.0105812122411,1.01053365079744,1.01048570399065))
REPRESENTATION_ITEM('')
);
#3135=(
BOUNDED_CURVE()
B_SPLINE_CURVE(2,(#20470,#20471,#20472),.UNSPECIFIED.,.F.,.F.)
B_SPLINE_CURVE_WITH_KNOTS((3,3),(-1.43398872568548,-1.42965690350654),
 .UNSPECIFIED.)
CURVE()
GEOMETRIC_REPRESENTATION_ITEM()
RATIONAL_B_SPLINE_CURVE((1.01048570399065,1.01053365079744,1.0105812122411))
REPRESENTATION_ITEM('')
);
#3136=(
BOUNDED_CURVE()
B_SPLINE_CURVE(2,(#20476,#20477,#20478),.UNSPECIFIED.,.F.,.F.)
B_SPLINE_CURVE_WITH_KNOTS((3,3),(-1.43398872568546,-1.42965690350652),
 .UNSPECIFIED.)
CURVE()
GEOMETRIC_REPRESENTATION_ITEM()
RATIONAL_B_SPLINE_CURVE((1.01048570399063,1.01053365079743,1.01058121224108))
REPRESENTATION_ITEM('')
);
#3137=(
BOUNDED_CURVE()
B_SPLINE_CURVE(2,(#20481,#20482,#20483),.UNSPECIFIED.,.F.,.F.)
B_SPLINE_CURVE_WITH_KNOTS((3,3),(-0.360391606906842,-0.356059784727902),
 .UNSPECIFIED.)
CURVE()
GEOMETRIC_REPRESENTATION_ITEM()
RATIONAL_B_SPLINE_CURVE((1.01058121224108,1.01053365079743,1.01048570399063))
REPRESENTATION_ITEM('')
);
#3267=LINE('',#19988,#4506);
#3268=LINE('',#19990,#4507);
#3269=LINE('',#19992,#4508);
#3270=LINE('',#19993,#4509);
#3271=LINE('',#19998,#4510);
#3272=LINE('',#20003,#4511);
#3273=LINE('',#20004,#4512);
#3274=LINE('',#20005,#4513);
#3275=LINE('',#20010,#4514);
#3276=LINE('',#20014,#4515);
#3277=LINE('',#20016,#4516);
#3278=LINE('',#20017,#4517);
#3279=LINE('',#20020,#4518);
#3280=LINE('',#20025,#4519);
#3281=LINE('',#20027,#4520);
#3282=LINE('',#20036,#4521);
#3283=LINE('',#20041,#4522);
#3284=LINE('',#20045,#4523);
#3285=LINE('',#20047,#4524);
#3286=LINE('',#20049,#4525);
#3287=LINE('',#20050,#4526);
#3288=LINE('',#20054,#4527);
#3289=LINE('',#20056,#4528);
#3290=LINE('',#20058,#4529);
#3291=LINE('',#20059,#4530);
#3292=LINE('',#20062,#4531);
#3293=LINE('',#20064,#4532);
#3294=LINE('',#20065,#4533);
#3295=LINE('',#20069,#4534);
#3296=LINE('',#20075,#4535);
#3297=LINE('',#20076,#4536);
#3298=LINE('',#20078,#4537);
#3299=LINE('',#20079,#4538);
#3300=LINE('',#20083,#4539);
#3301=LINE('',#20089,#4540);
#3302=LINE('',#20090,#4541);
#3303=LINE('',#20091,#4542);
#3304=LINE('',#20095,#4543);
#3305=LINE('',#20099,#4544);
#3306=LINE('',#20100,#4545);
#3307=LINE('',#20105,#4546);
#3308=LINE('',#20110,#4547);
#3309=LINE('',#20111,#4548);
#3310=LINE('',#20113,#4549);
#3311=LINE('',#20114,#4550);
#3312=LINE('',#20117,#4551);
#3313=LINE('',#20121,#4552);
#3314=LINE('',#20123,#4553);
#3315=LINE('',#20125,#4554);
#3316=LINE('',#20127,#4555);
#3317=LINE('',#20129,#4556);
#3318=LINE('',#20133,#4557);
#3319=LINE('',#20135,#4558);
#3320=LINE('',#20138,#4559);
#3321=LINE('',#20139,#4560);
#3322=LINE('',#20141,#4561);
#3323=LINE('',#20143,#4562);
#3324=LINE('',#20145,#4563);
#3325=LINE('',#20148,#4564);
#3326=LINE('',#20152,#4565);
#3327=LINE('',#20154,#4566);
#3328=LINE('',#20158,#4567);
#3329=LINE('',#20160,#4568);
#3330=LINE('',#20162,#4569);
#3331=LINE('',#20164,#4570);
#3332=LINE('',#20166,#4571);
#3333=LINE('',#20170,#4572);
#3334=LINE('',#20172,#4573);
#3335=LINE('',#20174,#4574);
#3336=LINE('',#20180,#4575);
#3337=LINE('',#20182,#4576);
#3338=LINE('',#20188,#4577);
#3339=LINE('',#20190,#4578);
#3340=LINE('',#20196,#4579);
#3341=LINE('',#20202,#4580);
#3342=LINE('',#20204,#4581);
#3343=LINE('',#20205,#4582);
#3344=LINE('',#20209,#4583);
#3345=LINE('',#20210,#4584);
#3346=LINE('',#20212,#4585);
#3347=LINE('',#20213,#4586);
#3348=LINE('',#20216,#4587);
#3349=LINE('',#20217,#4588);
#3350=LINE('',#20221,#4589);
#3351=LINE('',#20224,#4590);
#3352=LINE('',#20225,#4591);
#3353=LINE('',#20229,#4592);
#3354=LINE('',#20230,#4593);
#3355=LINE('',#20236,#4594);
#3356=LINE('',#20239,#4595);
#3357=LINE('',#20241,#4596);
#3358=LINE('',#20243,#4597);
#3359=LINE('',#20244,#4598);
#3360=LINE('',#20247,#4599);
#3361=LINE('',#20249,#4600);
#3362=LINE('',#20254,#4601);
#3363=LINE('',#20263,#4602);
#3364=LINE('',#20268,#4603);
#3365=LINE('',#20271,#4604);
#3366=LINE('',#20272,#4605);
#3367=LINE('',#20275,#4606);
#3368=LINE('',#20276,#4607);
#3369=LINE('',#20280,#4608);
#3370=LINE('',#20285,#4609);
#3371=LINE('',#20287,#4610);
#3372=LINE('',#20288,#4611);
#3373=LINE('',#20291,#4612);
#3374=LINE('',#20295,#4613);
#3375=LINE('',#20297,#4614);
#3376=LINE('',#20305,#4615);
#3377=LINE('',#20306,#4616);
#3378=LINE('',#20307,#4617);
#3379=LINE('',#20315,#4618);
#3380=LINE('',#20321,#4619);
#3381=LINE('',#20322,#4620);
#3382=LINE('',#20323,#4621);
#3383=LINE('',#20326,#4622);
#3384=LINE('',#20330,#4623);
#3385=LINE('',#20344,#4624);
#3386=LINE('',#20346,#4625);
#3387=LINE('',#20347,#4626);
#3388=LINE('',#20349,#4627);
#3389=LINE('',#20350,#4628);
#3390=LINE('',#20358,#4629);
#3391=LINE('',#20366,#4630);
#3392=LINE('',#20369,#4631);
#3393=LINE('',#20373,#4632);
#3394=LINE('',#20376,#4633);
#3395=LINE('',#20384,#4634);
#3396=LINE('',#20396,#4635);
#3397=LINE('',#20423,#4636);
#3398=LINE('',#20425,#4637);
#3399=LINE('',#20429,#4638);
#3400=LINE('',#20430,#4639);
#3401=LINE('',#20433,#4640);
#3402=LINE('',#20434,#4641);
#3403=LINE('',#20438,#4642);
#3404=LINE('',#20445,#4643);
#3405=LINE('',#20453,#4644);
#3406=LINE('',#20460,#4645);
#3407=LINE('',#20486,#4646);
#3408=LINE('',#20487,#4647);
#3409=LINE('',#20488,#4648);
#3410=LINE('',#20499,#4649);
#3411=LINE('',#20502,#4650);
#3412=LINE('',#20505,#4651);
#3413=LINE('',#20510,#4652);
#3414=LINE('',#20512,#4653);
#3415=LINE('',#20514,#4654);
#3416=LINE('',#20516,#4655);
#3417=LINE('',#20518,#4656);
#3418=LINE('',#20520,#4657);
#4506=VECTOR('',#16321,10.);
#4507=VECTOR('',#16322,10.);
#4508=VECTOR('',#16323,10.);
#4509=VECTOR('',#16324,10.);
#4510=VECTOR('',#16329,10.);
#4511=VECTOR('',#16334,10.);
#4512=VECTOR('',#16335,10.);
#4513=VECTOR('',#16336,10.);
#4514=VECTOR('',#16341,10.);
#4515=VECTOR('',#16346,10.);
#4516=VECTOR('',#16347,10.);
#4517=VECTOR('',#16348,10.);
#4518=VECTOR('',#16351,10.);
#4519=VECTOR('',#16352,10.);
#4520=VECTOR('',#16355,10.);
#4521=VECTOR('',#16360,10.);
#4522=VECTOR('',#16361,10.);
#4523=VECTOR('',#16364,10.);
#4524=VECTOR('',#16365,10.);
#4525=VECTOR('',#16366,10.);
#4526=VECTOR('',#16367,10.);
#4527=VECTOR('',#16370,10.);
#4528=VECTOR('',#16371,10.);
#4529=VECTOR('',#16372,10.);
#4530=VECTOR('',#16373,10.);
#4531=VECTOR('',#16376,10.);
#4532=VECTOR('',#16377,10.);
#4533=VECTOR('',#16378,10.);
#4534=VECTOR('',#16381,10.);
#4535=VECTOR('',#16388,10.);
#4536=VECTOR('',#16389,10.);
#4537=VECTOR('',#16390,10.);
#4538=VECTOR('',#16391,10.);
#4539=VECTOR('',#16394,10.);
#4540=VECTOR('',#16401,10.);
#4541=VECTOR('',#16402,10.);
#4542=VECTOR('',#16403,10.);
#4543=VECTOR('',#16406,10.);
#4544=VECTOR('',#16413,10.);
#4545=VECTOR('',#16414,10.);
#4546=VECTOR('',#16419,10.);
#4547=VECTOR('',#16424,10.);
#4548=VECTOR('',#16425,10.);
#4549=VECTOR('',#16426,10.);
#4550=VECTOR('',#16427,10.);
#4551=VECTOR('',#16430,10.);
#4552=VECTOR('',#16433,10.);
#4553=VECTOR('',#16434,10.);
#4554=VECTOR('',#16435,10.);
#4555=VECTOR('',#16436,10.);
#4556=VECTOR('',#16437,10.);
#4557=VECTOR('',#16440,10.);
#4558=VECTOR('',#16441,10.);
#4559=VECTOR('',#16444,10.);
#4560=VECTOR('',#16445,10.);
#4561=VECTOR('',#16448,10.);
#4562=VECTOR('',#16451,10.);
#4563=VECTOR('',#16454,10.);
#4564=VECTOR('',#16457,10.);
#4565=VECTOR('',#16460,10.);
#4566=VECTOR('',#16461,10.);
#4567=VECTOR('',#16464,10.);
#4568=VECTOR('',#16465,10.);
#4569=VECTOR('',#16466,10.);
#4570=VECTOR('',#16467,10.);
#4571=VECTOR('',#16468,10.);
#4572=VECTOR('',#16473,10.);
#4573=VECTOR('',#16474,10.);
#4574=VECTOR('',#16475,10.);
#4575=VECTOR('',#16478,10.);
#4576=VECTOR('',#16479,10.);
#4577=VECTOR('',#16482,10.);
#4578=VECTOR('',#16483,10.);
#4579=VECTOR('',#16484,10.);
#4580=VECTOR('',#16487,10.);
#4581=VECTOR('',#16488,10.);
#4582=VECTOR('',#16489,10.);
#4583=VECTOR('',#16492,10.);
#4584=VECTOR('',#16493,10.);
#4585=VECTOR('',#16494,10.);
#4586=VECTOR('',#16495,10.);
#4587=VECTOR('',#16498,10.);
#4588=VECTOR('',#16499,10.);
#4589=VECTOR('',#16504,10.);
#4590=VECTOR('',#16507,10.);
#4591=VECTOR('',#16508,10.);
#4592=VECTOR('',#16511,10.);
#4593=VECTOR('',#16512,10.);
#4594=VECTOR('',#16515,10.);
#4595=VECTOR('',#16518,10.);
#4596=VECTOR('',#16521,10.);
#4597=VECTOR('',#16524,10.);
#4598=VECTOR('',#16525,10.);
#4599=VECTOR('',#16528,10.);
#4600=VECTOR('',#16529,10.);
#4601=VECTOR('',#16532,10.);
#4602=VECTOR('',#16537,10.);
#4603=VECTOR('',#16540,10.);
#4604=VECTOR('',#16543,10.);
#4605=VECTOR('',#16544,10.);
#4606=VECTOR('',#16547,10.);
#4607=VECTOR('',#16548,10.);
#4608=VECTOR('',#16551,10.);
#4609=VECTOR('',#16558,10.);
#4610=VECTOR('',#16559,10.);
#4611=VECTOR('',#16560,10.);
#4612=VECTOR('',#16563,10.);
#4613=VECTOR('',#16570,10.);
#4614=VECTOR('',#16573,10.);
#4615=VECTOR('',#16582,10.);
#4616=VECTOR('',#16583,10.);
#4617=VECTOR('',#16584,10.);
#4618=VECTOR('',#16589,10.);
#4619=VECTOR('',#16596,10.);
#4620=VECTOR('',#16597,10.);
#4621=VECTOR('',#16598,10.);
#4622=VECTOR('',#16601,10.);
#4623=VECTOR('',#16608,10.);
#4624=VECTOR('',#16617,10.);
#4625=VECTOR('',#16618,10.);
#4626=VECTOR('',#16619,10.);
#4627=VECTOR('',#16622,10.);
#4628=VECTOR('',#16623,10.);
#4629=VECTOR('',#16630,10.);
#4630=VECTOR('',#16637,10.);
#4631=VECTOR('',#16638,10.);
#4632=VECTOR('',#16641,10.);
#4633=VECTOR('',#16646,10.);
#4634=VECTOR('',#16649,10.);
#4635=VECTOR('',#16652,10.);
#4636=VECTOR('',#16663,10.);
#4637=VECTOR('',#16664,10.);
#4638=VECTOR('',#16667,10.);
#4639=VECTOR('',#16668,10.);
#4640=VECTOR('',#16671,10.);
#4641=VECTOR('',#16672,10.);
#4642=VECTOR('',#16675,10.);
#4643=VECTOR('',#16676,10.);
#4644=VECTOR('',#16679,10.);
#4645=VECTOR('',#16680,10.);
#4646=VECTOR('',#16693,10.);
#4647=VECTOR('',#16694,10.);
#4648=VECTOR('',#16695,10.);
#4649=VECTOR('',#16714,10.);
#4650=VECTOR('',#16719,2.25);
#4651=VECTOR('',#16722,2.25);
#4652=VECTOR('',#16729,2.15);
#4653=VECTOR('',#16732,2.15);
#4654=VECTOR('',#16735,10.);
#4655=VECTOR('',#16738,10.);
#4656=VECTOR('',#16741,10.);
#4657=VECTOR('',#16744,10.);
#5741=VERTEX_POINT('',#19986);
#5742=VERTEX_POINT('',#19987);
#5743=VERTEX_POINT('',#19989);
#5744=VERTEX_POINT('',#19991);
#5745=VERTEX_POINT('',#19995);
#5746=VERTEX_POINT('',#19997);
#5747=VERTEX_POINT('',#20001);
#5748=VERTEX_POINT('',#20002);
#5749=VERTEX_POINT('',#20007);
#5750=VERTEX_POINT('',#20009);
#5751=VERTEX_POINT('',#20013);
#5752=VERTEX_POINT('',#20015);
#5753=VERTEX_POINT('',#20019);
#5754=VERTEX_POINT('',#20021);
#5755=VERTEX_POINT('',#20028);
#5756=VERTEX_POINT('',#20031);
#5757=VERTEX_POINT('',#20035);
#5758=VERTEX_POINT('',#20037);
#5759=VERTEX_POINT('',#20043);
#5760=VERTEX_POINT('',#20044);
#5761=VERTEX_POINT('',#20046);
#5762=VERTEX_POINT('',#20048);
#5763=VERTEX_POINT('',#20052);
#5764=VERTEX_POINT('',#20053);
#5765=VERTEX_POINT('',#20055);
#5766=VERTEX_POINT('',#20057);
#5767=VERTEX_POINT('',#20061);
#5768=VERTEX_POINT('',#20063);
#5769=VERTEX_POINT('',#20067);
#5770=VERTEX_POINT('',#20068);
#5771=VERTEX_POINT('',#20073);
#5772=VERTEX_POINT('',#20074);
#5773=VERTEX_POINT('',#20077);
#5774=VERTEX_POINT('',#20081);
#5775=VERTEX_POINT('',#20082);
#5776=VERTEX_POINT('',#20087);
#5777=VERTEX_POINT('',#20088);
#5778=VERTEX_POINT('',#20093);
#5779=VERTEX_POINT('',#20094);
#5780=VERTEX_POINT('',#20102);
#5781=VERTEX_POINT('',#20104);
#5782=VERTEX_POINT('',#20108);
#5783=VERTEX_POINT('',#20109);
#5784=VERTEX_POINT('',#20112);
#5785=VERTEX_POINT('',#20116);
#5786=VERTEX_POINT('',#20118);
#5787=VERTEX_POINT('',#20120);
#5788=VERTEX_POINT('',#20122);
#5789=VERTEX_POINT('',#20124);
#5790=VERTEX_POINT('',#20126);
#5791=VERTEX_POINT('',#20128);
#5792=VERTEX_POINT('',#20130);
#5793=VERTEX_POINT('',#20132);
#5794=VERTEX_POINT('',#20134);
#5795=VERTEX_POINT('',#20136);
#5796=VERTEX_POINT('',#20147);
#5797=VERTEX_POINT('',#20149);
#5798=VERTEX_POINT('',#20151);
#5799=VERTEX_POINT('',#20153);
#5800=VERTEX_POINT('',#20155);
#5801=VERTEX_POINT('',#20157);
#5802=VERTEX_POINT('',#20159);
#5803=VERTEX_POINT('',#20161);
#5804=VERTEX_POINT('',#20163);
#5805=VERTEX_POINT('',#20165);
#5806=VERTEX_POINT('',#20169);
#5807=VERTEX_POINT('',#20171);
#5808=VERTEX_POINT('',#20173);
#5809=VERTEX_POINT('',#20179);
#5810=VERTEX_POINT('',#20181);
#5811=VERTEX_POINT('',#20187);
#5812=VERTEX_POINT('',#20189);
#5813=VERTEX_POINT('',#20191);
#5814=VERTEX_POINT('',#20195);
#5815=VERTEX_POINT('',#20201);
#5816=VERTEX_POINT('',#20203);
#5817=VERTEX_POINT('',#20207);
#5818=VERTEX_POINT('',#20208);
#5819=VERTEX_POINT('',#20211);
#5820=VERTEX_POINT('',#20215);
#5821=VERTEX_POINT('',#20219);
#5822=VERTEX_POINT('',#20223);
#5823=VERTEX_POINT('',#20227);
#5824=VERTEX_POINT('',#20228);
#5825=VERTEX_POINT('',#20235);
#5826=VERTEX_POINT('',#20237);
#5827=VERTEX_POINT('',#20246);
#5828=VERTEX_POINT('',#20248);
#5829=VERTEX_POINT('',#20255);
#5830=VERTEX_POINT('',#20258);
#5831=VERTEX_POINT('',#20262);
#5832=VERTEX_POINT('',#20270);
#5833=VERTEX_POINT('',#20274);
#5834=VERTEX_POINT('',#20278);
#5835=VERTEX_POINT('',#20279);
#5836=VERTEX_POINT('',#20284);
#5837=VERTEX_POINT('',#20286);
#5838=VERTEX_POINT('',#20290);
#5839=VERTEX_POINT('',#20298);
#5840=VERTEX_POINT('',#20301);
#5841=VERTEX_POINT('',#20304);
#5842=VERTEX_POINT('',#20313);
#5843=VERTEX_POINT('',#20314);
#5844=VERTEX_POINT('',#20319);
#5845=VERTEX_POINT('',#20320);
#5846=VERTEX_POINT('',#20325);
#5847=VERTEX_POINT('',#20332);
#5848=VERTEX_POINT('',#20339);
#5849=VERTEX_POINT('',#20343);
#5850=VERTEX_POINT('',#20345);
#5851=VERTEX_POINT('',#20352);
#5852=VERTEX_POINT('',#20360);
#5853=VERTEX_POINT('',#20367);
#5854=VERTEX_POINT('',#20368);
#5855=VERTEX_POINT('',#20370);
#5856=VERTEX_POINT('',#20372);
#5857=VERTEX_POINT('',#20378);
#5858=VERTEX_POINT('',#20383);
#5859=VERTEX_POINT('',#20390);
#5860=VERTEX_POINT('',#20395);
#5861=VERTEX_POINT('',#20402);
#5862=VERTEX_POINT('',#20403);
#5863=VERTEX_POINT('',#20412);
#5864=VERTEX_POINT('',#20416);
#5865=VERTEX_POINT('',#20422);
#5866=VERTEX_POINT('',#20424);
#5867=VERTEX_POINT('',#20426);
#5868=VERTEX_POINT('',#20428);
#5869=VERTEX_POINT('',#20432);
#5870=VERTEX_POINT('',#20436);
#5871=VERTEX_POINT('',#20437);
#5872=VERTEX_POINT('',#20439);
#5873=VERTEX_POINT('',#20444);
#5874=VERTEX_POINT('',#20451);
#5875=VERTEX_POINT('',#20452);
#5876=VERTEX_POINT('',#20454);
#5877=VERTEX_POINT('',#20459);
#5878=VERTEX_POINT('',#20475);
#5879=VERTEX_POINT('',#20479);
#5880=VERTEX_POINT('',#20485);
#5881=VERTEX_POINT('',#20495);
#5882=VERTEX_POINT('',#20504);
#5883=VERTEX_POINT('',#20508);
#7127=EDGE_CURVE('',#5741,#5742,#3267,.F.);
#7128=EDGE_CURVE('',#5742,#5743,#3268,.T.);
#7129=EDGE_CURVE('',#5743,#5744,#3269,.T.);
#7130=EDGE_CURVE('',#5744,#5741,#3270,.T.);
#7131=EDGE_CURVE('',#5743,#5745,#971,.T.);
#7132=EDGE_CURVE('',#5745,#5746,#3271,.T.);
#7133=EDGE_CURVE('',#5746,#5744,#972,.T.);
#7134=EDGE_CURVE('',#5747,#5748,#3272,.T.);
#7135=EDGE_CURVE('',#5748,#5746,#3273,.T.);
#7136=EDGE_CURVE('',#5745,#5747,#3274,.T.);
#7137=EDGE_CURVE('',#5747,#5749,#973,.T.);
#7138=EDGE_CURVE('',#5749,#5750,#3275,.T.);
#7139=EDGE_CURVE('',#5750,#5748,#974,.T.);
#7140=EDGE_CURVE('',#5751,#5750,#3276,.T.);
#7141=EDGE_CURVE('',#5749,#5752,#3277,.T.);
#7142=EDGE_CURVE('',#5752,#5751,#3278,.T.);
#7143=EDGE_CURVE('',#5752,#5753,#3279,.T.);
#7144=EDGE_CURVE('',#5753,#5754,#3114,.F.);
#7145=EDGE_CURVE('',#5754,#5751,#3280,.T.);
#7146=EDGE_CURVE('',#5741,#5751,#3281,.T.);
#7147=EDGE_CURVE('',#5755,#5755,#975,.T.);
#7148=EDGE_CURVE('',#5756,#5754,#3115,.F.);
#7149=EDGE_CURVE('',#5757,#5756,#3282,.T.);
#7150=EDGE_CURVE('',#5758,#5757,#3116,.F.);
#7151=EDGE_CURVE('',#5741,#5758,#3283,.T.);
#7152=EDGE_CURVE('',#5759,#5760,#3284,.T.);
#7153=EDGE_CURVE('',#5760,#5761,#3285,.T.);
#7154=EDGE_CURVE('',#5761,#5762,#3286,.T.);
#7155=EDGE_CURVE('',#5762,#5759,#3287,.T.);
#7156=EDGE_CURVE('',#5763,#5764,#3288,.T.);
#7157=EDGE_CURVE('',#5764,#5765,#3289,.T.);
#7158=EDGE_CURVE('',#5765,#5766,#3290,.T.);
#7159=EDGE_CURVE('',#5766,#5763,#3291,.T.);
#7160=EDGE_CURVE('',#5766,#5767,#3292,.T.);
#7161=EDGE_CURVE('',#5767,#5768,#3293,.T.);
#7162=EDGE_CURVE('',#5768,#5763,#3294,.T.);
#7163=EDGE_CURVE('',#5769,#5770,#3295,.T.);
#7164=EDGE_CURVE('',#5770,#5768,#976,.T.);
#7165=EDGE_CURVE('',#5767,#5769,#977,.T.);
#7166=EDGE_CURVE('',#5771,#5772,#3296,.T.);
#7167=EDGE_CURVE('',#5772,#5770,#3297,.T.);
#7168=EDGE_CURVE('',#5769,#5773,#3298,.T.);
#7169=EDGE_CURVE('',#5773,#5771,#3299,.T.);
#7170=EDGE_CURVE('',#5774,#5775,#3300,.T.);
#7171=EDGE_CURVE('',#5775,#5765,#978,.T.);
#7172=EDGE_CURVE('',#5764,#5774,#979,.T.);
#7173=EDGE_CURVE('',#5776,#5777,#3301,.T.);
#7174=EDGE_CURVE('',#5777,#5775,#3302,.T.);
#7175=EDGE_CURVE('',#5774,#5776,#3303,.T.);
#7176=EDGE_CURVE('',#5778,#5779,#3304,.T.);
#7177=EDGE_CURVE('',#5779,#5777,#980,.T.);
#7178=EDGE_CURVE('',#5776,#5778,#981,.T.);
#7179=EDGE_CURVE('',#5762,#5779,#3305,.T.);
#7180=EDGE_CURVE('',#5778,#5759,#3306,.T.);
#7181=EDGE_CURVE('',#5760,#5780,#982,.T.);
#7182=EDGE_CURVE('',#5780,#5781,#3307,.T.);
#7183=EDGE_CURVE('',#5781,#5761,#983,.T.);
#7184=EDGE_CURVE('',#5782,#5783,#3308,.T.);
#7185=EDGE_CURVE('',#5783,#5781,#3309,.T.);
#7186=EDGE_CURVE('',#5780,#5784,#3310,.T.);
#7187=EDGE_CURVE('',#5784,#5782,#3311,.T.);
#7188=EDGE_CURVE('',#5785,#5742,#3312,.T.);
#7189=EDGE_CURVE('',#5786,#5785,#984,.T.);
#7190=EDGE_CURVE('',#5787,#5786,#3313,.T.);
#7191=EDGE_CURVE('',#5788,#5787,#3314,.T.);
#7192=EDGE_CURVE('',#5789,#5788,#3315,.T.);
#7193=EDGE_CURVE('',#5790,#5789,#3316,.T.);
#7194=EDGE_CURVE('',#5791,#5790,#3317,.T.);
#7195=EDGE_CURVE('',#5792,#5791,#985,.T.);
#7196=EDGE_CURVE('',#5793,#5792,#3318,.T.);
#7197=EDGE_CURVE('',#5794,#5793,#3319,.T.);
#7198=EDGE_CURVE('',#5795,#5794,#986,.T.);
#7199=EDGE_CURVE('',#5773,#5795,#3320,.T.);
#7200=EDGE_CURVE('',#5743,#5765,#3321,.T.);
#7201=EDGE_CURVE('',#5775,#5745,#3322,.T.);
#7202=EDGE_CURVE('',#5747,#5777,#3323,.T.);
#7203=EDGE_CURVE('',#5779,#5749,#3324,.T.);
#7204=EDGE_CURVE('',#5796,#5783,#3325,.T.);
#7205=EDGE_CURVE('',#5797,#5796,#987,.T.);
#7206=EDGE_CURVE('',#5798,#5797,#3326,.T.);
#7207=EDGE_CURVE('',#5799,#5798,#3327,.T.);
#7208=EDGE_CURVE('',#5800,#5799,#988,.T.);
#7209=EDGE_CURVE('',#5801,#5800,#3328,.T.);
#7210=EDGE_CURVE('',#5802,#5801,#3329,.T.);
#7211=EDGE_CURVE('',#5803,#5802,#3330,.T.);
#7212=EDGE_CURVE('',#5804,#5803,#3331,.T.);
#7213=EDGE_CURVE('',#5805,#5804,#3332,.T.);
#7214=EDGE_CURVE('',#5753,#5805,#989,.T.);
#7215=EDGE_CURVE('',#5806,#5782,#3333,.T.);
#7216=EDGE_CURVE('',#5806,#5807,#3334,.T.);
#7217=EDGE_CURVE('',#5807,#5808,#3335,.T.);
#7218=EDGE_CURVE('',#5808,#5796,#3117,.T.);
#7219=EDGE_CURVE('',#5804,#5809,#3336,.F.);
#7220=EDGE_CURVE('',#5809,#5810,#3337,.T.);
#7221=EDGE_CURVE('',#5810,#5805,#3118,.F.);
#7222=EDGE_CURVE('',#5811,#5809,#3338,.T.);
#7223=EDGE_CURVE('',#5812,#5811,#3339,.T.);
#7224=EDGE_CURVE('',#5813,#5812,#3119,.F.);
#7225=EDGE_CURVE('',#5813,#5814,#3340,.T.);
#7226=EDGE_CURVE('',#5810,#5814,#3120,.F.);
#7227=EDGE_CURVE('',#5815,#5798,#3341,.T.);
#7228=EDGE_CURVE('',#5816,#5815,#3342,.T.);
#7229=EDGE_CURVE('',#5798,#5816,#3343,.T.);
#7230=EDGE_CURVE('',#5817,#5818,#3344,.T.);
#7231=EDGE_CURVE('',#5818,#5816,#3345,.T.);
#7232=EDGE_CURVE('',#5815,#5819,#3346,.T.);
#7233=EDGE_CURVE('',#5819,#5817,#3347,.T.);
#7234=EDGE_CURVE('',#5820,#5799,#3348,.T.);
#7235=EDGE_CURVE('',#5816,#5820,#3349,.T.);
#7236=EDGE_CURVE('',#5820,#5821,#990,.T.);
#7237=EDGE_CURVE('',#5821,#5800,#3350,.T.);
#7238=EDGE_CURVE('',#5822,#5801,#3351,.F.);
#7239=EDGE_CURVE('',#5821,#5822,#3352,.T.);
#7240=EDGE_CURVE('',#5823,#5824,#3353,.T.);
#7241=EDGE_CURVE('',#5824,#5815,#3354,.T.);
#7242=EDGE_CURVE('',#5797,#5823,#3121,.T.);
#7243=EDGE_CURVE('',#5820,#5825,#3355,.T.);
#7244=EDGE_CURVE('',#5826,#5825,#991,.T.);
#7245=EDGE_CURVE('',#5826,#5821,#3356,.T.);
#7246=EDGE_CURVE('',#5825,#5818,#3357,.T.);
#7247=EDGE_CURVE('',#5793,#5817,#3358,.T.);
#7248=EDGE_CURVE('',#5792,#5825,#3359,.T.);
#7249=EDGE_CURVE('',#5819,#5827,#3360,.T.);
#7250=EDGE_CURVE('',#5827,#5828,#3361,.T.);
#7251=EDGE_CURVE('',#5828,#5794,#3122,.T.);
#7252=EDGE_CURVE('',#5827,#5824,#3362,.T.);
#7253=EDGE_CURVE('',#5829,#5829,#992,.T.);
#7254=EDGE_CURVE('',#5823,#5830,#3123,.T.);
#7255=EDGE_CURVE('',#5830,#5831,#3363,.T.);
#7256=EDGE_CURVE('',#5831,#5828,#3124,.T.);
#7257=EDGE_CURVE('',#5791,#5826,#3364,.T.);
#7258=EDGE_CURVE('',#5832,#5826,#3365,.T.);
#7259=EDGE_CURVE('',#5790,#5832,#3366,.T.);
#7260=EDGE_CURVE('',#5822,#5833,#3367,.T.);
#7261=EDGE_CURVE('',#5833,#5802,#3368,.T.);
#7262=EDGE_CURVE('',#5834,#5835,#3369,.T.);
#7263=EDGE_CURVE('',#5835,#5802,#993,.T.);
#7264=EDGE_CURVE('',#5833,#5834,#994,.T.);
#7265=EDGE_CURVE('',#5834,#5836,#3370,.T.);
#7266=EDGE_CURVE('',#5836,#5837,#3371,.T.);
#7267=EDGE_CURVE('',#5837,#5835,#3372,.T.);
#7268=EDGE_CURVE('',#5838,#5789,#3373,.T.);
#7269=EDGE_CURVE('',#5789,#5837,#995,.T.);
#7270=EDGE_CURVE('',#5836,#5838,#996,.T.);
#7271=EDGE_CURVE('',#5838,#5832,#3374,.T.);
#7272=EDGE_CURVE('',#5832,#5822,#3375,.T.);
#7273=EDGE_CURVE('',#5839,#5839,#997,.T.);
#7274=EDGE_CURVE('',#5840,#5840,#998,.T.);
#7275=EDGE_CURVE('',#5811,#5841,#3376,.T.);
#7276=EDGE_CURVE('',#5841,#5788,#3377,.T.);
#7277=EDGE_CURVE('',#5787,#5811,#3378,.T.);
#7278=EDGE_CURVE('',#5786,#5812,#3125,.F.);
#7279=EDGE_CURVE('',#5842,#5843,#3379,.T.);
#7280=EDGE_CURVE('',#5843,#5788,#999,.T.);
#7281=EDGE_CURVE('',#5841,#5842,#1000,.T.);
#7282=EDGE_CURVE('',#5844,#5845,#3380,.T.);
#7283=EDGE_CURVE('',#5845,#5843,#3381,.T.);
#7284=EDGE_CURVE('',#5842,#5844,#3382,.T.);
#7285=EDGE_CURVE('',#5846,#5803,#3383,.T.);
#7286=EDGE_CURVE('',#5803,#5845,#1001,.T.);
#7287=EDGE_CURVE('',#5844,#5846,#1002,.T.);
#7288=EDGE_CURVE('',#5846,#5809,#3384,.T.);
#7289=EDGE_CURVE('',#5847,#5847,#1003,.T.);
#7290=EDGE_CURVE('',#5758,#5785,#3126,.F.);
#7291=EDGE_CURVE('',#5795,#5848,#3127,.T.);
#7292=EDGE_CURVE('',#5848,#5849,#3385,.T.);
#7293=EDGE_CURVE('',#5849,#5850,#3386,.T.);
#7294=EDGE_CURVE('',#5850,#5771,#3387,.T.);
#7295=EDGE_CURVE('',#5850,#5806,#3388,.T.);
#7296=EDGE_CURVE('',#5784,#5772,#3389,.T.);
#7297=EDGE_CURVE('',#5831,#5851,#1004,.T.);
#7298=EDGE_CURVE('',#5848,#5851,#3128,.T.);
#7299=EDGE_CURVE('',#5770,#5780,#3390,.T.);
#7300=EDGE_CURVE('',#5852,#5808,#3129,.T.);
#7301=EDGE_CURVE('',#5852,#5830,#1005,.T.);
#7302=EDGE_CURVE('',#5851,#5852,#3391,.T.);
#7303=EDGE_CURVE('',#5853,#5854,#3392,.T.);
#7304=EDGE_CURVE('',#5855,#5853,#1006,.T.);
#7305=EDGE_CURVE('',#5856,#5855,#3393,.T.);
#7306=EDGE_CURVE('',#5854,#5856,#1007,.T.);
#7307=EDGE_CURVE('',#5807,#5849,#3394,.T.);
#7308=EDGE_CURVE('',#5855,#5857,#120,.T.);
#7309=EDGE_CURVE('',#5857,#5858,#3395,.T.);
#7310=EDGE_CURVE('',#5858,#5856,#121,.T.);
#7311=EDGE_CURVE('',#5854,#5859,#122,.T.);
#7312=EDGE_CURVE('',#5859,#5860,#3396,.T.);
#7313=EDGE_CURVE('',#5860,#5853,#123,.T.);
#7314=EDGE_CURVE('',#5861,#5862,#1008,.T.);
#7315=EDGE_CURVE('',#5862,#5859,#3130,.T.);
#7316=EDGE_CURVE('',#5858,#5861,#3131,.T.);
#7317=EDGE_CURVE('',#5860,#5863,#3132,.T.);
#7318=EDGE_CURVE('',#5863,#5864,#1009,.T.);
#7319=EDGE_CURVE('',#5864,#5857,#3133,.T.);
#7320=EDGE_CURVE('',#5865,#5863,#3397,.T.);
#7321=EDGE_CURVE('',#5866,#5865,#3398,.T.);
#7322=EDGE_CURVE('',#5867,#5866,#1010,.T.);
#7323=EDGE_CURVE('',#5868,#5867,#3399,.T.);
#7324=EDGE_CURVE('',#5864,#5868,#3400,.T.);
#7325=EDGE_CURVE('',#5862,#5869,#3401,.T.);
#7326=EDGE_CURVE('',#5865,#5869,#3402,.T.);
#7327=EDGE_CURVE('',#5870,#5871,#3403,.T.);
#7328=EDGE_CURVE('',#5871,#5872,#124,.T.);
#7329=EDGE_CURVE('',#5872,#5873,#3404,.T.);
#7330=EDGE_CURVE('',#5873,#5870,#125,.T.);
#7331=EDGE_CURVE('',#5874,#5875,#3405,.T.);
#7332=EDGE_CURVE('',#5875,#5876,#126,.T.);
#7333=EDGE_CURVE('',#5876,#5877,#3406,.T.);
#7334=EDGE_CURVE('',#5877,#5874,#127,.T.);
#7335=EDGE_CURVE('',#5866,#5876,#3134,.T.);
#7336=EDGE_CURVE('',#5875,#5870,#1011,.T.);
#7337=EDGE_CURVE('',#5873,#5867,#3135,.T.);
#7338=EDGE_CURVE('',#5871,#5874,#1012,.T.);
#7339=EDGE_CURVE('',#5877,#5878,#3136,.T.);
#7340=EDGE_CURVE('',#5878,#5879,#1013,.T.);
#7341=EDGE_CURVE('',#5879,#5872,#3137,.T.);
#7342=EDGE_CURVE('',#5880,#5861,#3407,.T.);
#7343=EDGE_CURVE('',#5879,#5880,#3408,.T.);
#7344=EDGE_CURVE('',#5869,#5878,#3409,.T.);
#7345=EDGE_CURVE('',#5814,#5756,#1014,.T.);
#7346=EDGE_CURVE('',#5757,#5813,#1015,.T.);
#7347=EDGE_CURVE('',#5881,#5881,#1016,.T.);
#7348=EDGE_CURVE('',#5868,#5880,#3410,.T.);
#7349=EDGE_CURVE('',#5829,#5839,#3411,.T.);
#7350=EDGE_CURVE('',#5881,#5882,#3412,.T.);
#7351=EDGE_CURVE('',#5882,#5882,#1017,.T.);
#7352=EDGE_CURVE('',#5883,#5883,#1018,.T.);
#7353=EDGE_CURVE('',#5883,#5755,#3413,.T.);
#7354=EDGE_CURVE('',#5840,#5847,#3414,.T.);
#7355=EDGE_CURVE('',#5843,#5837,#3415,.T.);
#7356=EDGE_CURVE('',#5835,#5845,#3416,.T.);
#7357=EDGE_CURVE('',#5760,#5768,#3417,.T.);
#7358=EDGE_CURVE('',#5763,#5759,#3418,.T.);
#9371=ORIENTED_EDGE('',*,*,#7127,.T.);
#9372=ORIENTED_EDGE('',*,*,#7128,.T.);
#9373=ORIENTED_EDGE('',*,*,#7129,.T.);
#9374=ORIENTED_EDGE('',*,*,#7130,.T.);
#9375=ORIENTED_EDGE('',*,*,#7129,.F.);
#9376=ORIENTED_EDGE('',*,*,#7131,.T.);
#9377=ORIENTED_EDGE('',*,*,#7132,.T.);
#9378=ORIENTED_EDGE('',*,*,#7133,.T.);
#9379=ORIENTED_EDGE('',*,*,#7134,.T.);
#9380=ORIENTED_EDGE('',*,*,#7135,.T.);
#9381=ORIENTED_EDGE('',*,*,#7132,.F.);
#9382=ORIENTED_EDGE('',*,*,#7136,.T.);
#9383=ORIENTED_EDGE('',*,*,#7134,.F.);
#9384=ORIENTED_EDGE('',*,*,#7137,.T.);
#9385=ORIENTED_EDGE('',*,*,#7138,.T.);
#9386=ORIENTED_EDGE('',*,*,#7139,.T.);
#9387=ORIENTED_EDGE('',*,*,#7140,.T.);
#9388=ORIENTED_EDGE('',*,*,#7138,.F.);
#9389=ORIENTED_EDGE('',*,*,#7141,.T.);
#9390=ORIENTED_EDGE('',*,*,#7142,.T.);
#9391=ORIENTED_EDGE('',*,*,#7143,.T.);
#9392=ORIENTED_EDGE('',*,*,#7144,.T.);
#9393=ORIENTED_EDGE('',*,*,#7145,.T.);
#9394=ORIENTED_EDGE('',*,*,#7142,.F.);
#9395=ORIENTED_EDGE('',*,*,#7130,.F.);
#9396=ORIENTED_EDGE('',*,*,#7133,.F.);
#9397=ORIENTED_EDGE('',*,*,#7135,.F.);
#9398=ORIENTED_EDGE('',*,*,#7139,.F.);
#9399=ORIENTED_EDGE('',*,*,#7140,.F.);
#9400=ORIENTED_EDGE('',*,*,#7146,.F.);
#9401=ORIENTED_EDGE('',*,*,#7147,.T.);
#9402=ORIENTED_EDGE('',*,*,#7145,.F.);
#9403=ORIENTED_EDGE('',*,*,#7148,.F.);
#9404=ORIENTED_EDGE('',*,*,#7149,.F.);
#9405=ORIENTED_EDGE('',*,*,#7150,.F.);
#9406=ORIENTED_EDGE('',*,*,#7151,.F.);
#9407=ORIENTED_EDGE('',*,*,#7146,.T.);
#9408=ORIENTED_EDGE('',*,*,#7152,.T.);
#9409=ORIENTED_EDGE('',*,*,#7153,.T.);
#9410=ORIENTED_EDGE('',*,*,#7154,.T.);
#9411=ORIENTED_EDGE('',*,*,#7155,.T.);
#9412=ORIENTED_EDGE('',*,*,#7156,.T.);
#9413=ORIENTED_EDGE('',*,*,#7157,.T.);
#9414=ORIENTED_EDGE('',*,*,#7158,.T.);
#9415=ORIENTED_EDGE('',*,*,#7159,.T.);
#9416=ORIENTED_EDGE('',*,*,#7160,.T.);
#9417=ORIENTED_EDGE('',*,*,#7161,.T.);
#9418=ORIENTED_EDGE('',*,*,#7162,.T.);
#9419=ORIENTED_EDGE('',*,*,#7159,.F.);
#9420=ORIENTED_EDGE('',*,*,#7163,.T.);
#9421=ORIENTED_EDGE('',*,*,#7164,.T.);
#9422=ORIENTED_EDGE('',*,*,#7161,.F.);
#9423=ORIENTED_EDGE('',*,*,#7165,.T.);
#9424=ORIENTED_EDGE('',*,*,#7166,.T.);
#9425=ORIENTED_EDGE('',*,*,#7167,.T.);
#9426=ORIENTED_EDGE('',*,*,#7163,.F.);
#9427=ORIENTED_EDGE('',*,*,#7168,.T.);
#9428=ORIENTED_EDGE('',*,*,#7169,.T.);
#9429=ORIENTED_EDGE('',*,*,#7170,.T.);
#9430=ORIENTED_EDGE('',*,*,#7171,.T.);
#9431=ORIENTED_EDGE('',*,*,#7157,.F.);
#9432=ORIENTED_EDGE('',*,*,#7172,.T.);
#9433=ORIENTED_EDGE('',*,*,#7173,.T.);
#9434=ORIENTED_EDGE('',*,*,#7174,.T.);
#9435=ORIENTED_EDGE('',*,*,#7170,.F.);
#9436=ORIENTED_EDGE('',*,*,#7175,.T.);
#9437=ORIENTED_EDGE('',*,*,#7176,.T.);
#9438=ORIENTED_EDGE('',*,*,#7177,.T.);
#9439=ORIENTED_EDGE('',*,*,#7173,.F.);
#9440=ORIENTED_EDGE('',*,*,#7178,.T.);
#9441=ORIENTED_EDGE('',*,*,#7179,.T.);
#9442=ORIENTED_EDGE('',*,*,#7176,.F.);
#9443=ORIENTED_EDGE('',*,*,#7180,.T.);
#9444=ORIENTED_EDGE('',*,*,#7155,.F.);
#9445=ORIENTED_EDGE('',*,*,#7153,.F.);
#9446=ORIENTED_EDGE('',*,*,#7181,.T.);
#9447=ORIENTED_EDGE('',*,*,#7182,.T.);
#9448=ORIENTED_EDGE('',*,*,#7183,.T.);
#9449=ORIENTED_EDGE('',*,*,#7184,.T.);
#9450=ORIENTED_EDGE('',*,*,#7185,.T.);
#9451=ORIENTED_EDGE('',*,*,#7182,.F.);
#9452=ORIENTED_EDGE('',*,*,#7186,.T.);
#9453=ORIENTED_EDGE('',*,*,#7187,.T.);
#9454=ORIENTED_EDGE('',*,*,#7188,.F.);
#9455=ORIENTED_EDGE('',*,*,#7189,.F.);
#9456=ORIENTED_EDGE('',*,*,#7190,.F.);
#9457=ORIENTED_EDGE('',*,*,#7191,.F.);
#9458=ORIENTED_EDGE('',*,*,#7192,.F.);
#9459=ORIENTED_EDGE('',*,*,#7193,.F.);
#9460=ORIENTED_EDGE('',*,*,#7194,.F.);
#9461=ORIENTED_EDGE('',*,*,#7195,.F.);
#9462=ORIENTED_EDGE('',*,*,#7196,.F.);
#9463=ORIENTED_EDGE('',*,*,#7197,.F.);
#9464=ORIENTED_EDGE('',*,*,#7198,.F.);
#9465=ORIENTED_EDGE('',*,*,#7199,.F.);
#9466=ORIENTED_EDGE('',*,*,#7168,.F.);
#9467=ORIENTED_EDGE('',*,*,#7165,.F.);
#9468=ORIENTED_EDGE('',*,*,#7160,.F.);
#9469=ORIENTED_EDGE('',*,*,#7158,.F.);
#9470=ORIENTED_EDGE('',*,*,#7200,.F.);
#9471=ORIENTED_EDGE('',*,*,#7128,.F.);
#9472=ORIENTED_EDGE('',*,*,#7131,.F.);
#9473=ORIENTED_EDGE('',*,*,#7200,.T.);
#9474=ORIENTED_EDGE('',*,*,#7171,.F.);
#9475=ORIENTED_EDGE('',*,*,#7201,.T.);
#9476=ORIENTED_EDGE('',*,*,#7136,.F.);
#9477=ORIENTED_EDGE('',*,*,#7201,.F.);
#9478=ORIENTED_EDGE('',*,*,#7174,.F.);
#9479=ORIENTED_EDGE('',*,*,#7202,.F.);
#9480=ORIENTED_EDGE('',*,*,#7137,.F.);
#9481=ORIENTED_EDGE('',*,*,#7202,.T.);
#9482=ORIENTED_EDGE('',*,*,#7177,.F.);
#9483=ORIENTED_EDGE('',*,*,#7203,.T.);
#9484=ORIENTED_EDGE('',*,*,#7141,.F.);
#9485=ORIENTED_EDGE('',*,*,#7203,.F.);
#9486=ORIENTED_EDGE('',*,*,#7179,.F.);
#9487=ORIENTED_EDGE('',*,*,#7154,.F.);
#9488=ORIENTED_EDGE('',*,*,#7183,.F.);
#9489=ORIENTED_EDGE('',*,*,#7185,.F.);
#9490=ORIENTED_EDGE('',*,*,#7204,.F.);
#9491=ORIENTED_EDGE('',*,*,#7205,.F.);
#9492=ORIENTED_EDGE('',*,*,#7206,.F.);
#9493=ORIENTED_EDGE('',*,*,#7207,.F.);
#9494=ORIENTED_EDGE('',*,*,#7208,.F.);
#9495=ORIENTED_EDGE('',*,*,#7209,.F.);
#9496=ORIENTED_EDGE('',*,*,#7210,.F.);
#9497=ORIENTED_EDGE('',*,*,#7211,.F.);
#9498=ORIENTED_EDGE('',*,*,#7212,.F.);
#9499=ORIENTED_EDGE('',*,*,#7213,.F.);
#9500=ORIENTED_EDGE('',*,*,#7214,.F.);
#9501=ORIENTED_EDGE('',*,*,#7143,.F.);
#9502=ORIENTED_EDGE('',*,*,#7184,.F.);
#9503=ORIENTED_EDGE('',*,*,#7215,.F.);
#9504=ORIENTED_EDGE('',*,*,#7216,.T.);
#9505=ORIENTED_EDGE('',*,*,#7217,.T.);
#9506=ORIENTED_EDGE('',*,*,#7218,.T.);
#9507=ORIENTED_EDGE('',*,*,#7204,.T.);
#9508=ORIENTED_EDGE('',*,*,#7219,.T.);
#9509=ORIENTED_EDGE('',*,*,#7220,.T.);
#9510=ORIENTED_EDGE('',*,*,#7221,.T.);
#9511=ORIENTED_EDGE('',*,*,#7213,.T.);
#9512=ORIENTED_EDGE('',*,*,#7220,.F.);
#9513=ORIENTED_EDGE('',*,*,#7222,.F.);
#9514=ORIENTED_EDGE('',*,*,#7223,.F.);
#9515=ORIENTED_EDGE('',*,*,#7224,.F.);
#9516=ORIENTED_EDGE('',*,*,#7225,.T.);
#9517=ORIENTED_EDGE('',*,*,#7226,.F.);
#9518=ORIENTED_EDGE('',*,*,#7227,.F.);
#9519=ORIENTED_EDGE('',*,*,#7228,.F.);
#9520=ORIENTED_EDGE('',*,*,#7229,.F.);
#9521=ORIENTED_EDGE('',*,*,#7230,.T.);
#9522=ORIENTED_EDGE('',*,*,#7231,.T.);
#9523=ORIENTED_EDGE('',*,*,#7228,.T.);
#9524=ORIENTED_EDGE('',*,*,#7232,.T.);
#9525=ORIENTED_EDGE('',*,*,#7233,.T.);
#9526=ORIENTED_EDGE('',*,*,#7234,.T.);
#9527=ORIENTED_EDGE('',*,*,#7207,.T.);
#9528=ORIENTED_EDGE('',*,*,#7229,.T.);
#9529=ORIENTED_EDGE('',*,*,#7235,.T.);
#9530=ORIENTED_EDGE('',*,*,#7234,.F.);
#9531=ORIENTED_EDGE('',*,*,#7236,.T.);
#9532=ORIENTED_EDGE('',*,*,#7237,.T.);
#9533=ORIENTED_EDGE('',*,*,#7208,.T.);
#9534=ORIENTED_EDGE('',*,*,#7238,.T.);
#9535=ORIENTED_EDGE('',*,*,#7209,.T.);
#9536=ORIENTED_EDGE('',*,*,#7237,.F.);
#9537=ORIENTED_EDGE('',*,*,#7239,.T.);
#9538=ORIENTED_EDGE('',*,*,#7240,.T.);
#9539=ORIENTED_EDGE('',*,*,#7241,.T.);
#9540=ORIENTED_EDGE('',*,*,#7227,.T.);
#9541=ORIENTED_EDGE('',*,*,#7206,.T.);
#9542=ORIENTED_EDGE('',*,*,#7242,.T.);
#9543=ORIENTED_EDGE('',*,*,#7236,.F.);
#9544=ORIENTED_EDGE('',*,*,#7243,.T.);
#9545=ORIENTED_EDGE('',*,*,#7244,.F.);
#9546=ORIENTED_EDGE('',*,*,#7245,.T.);
#9547=ORIENTED_EDGE('',*,*,#7235,.F.);
#9548=ORIENTED_EDGE('',*,*,#7231,.F.);
#9549=ORIENTED_EDGE('',*,*,#7246,.F.);
#9550=ORIENTED_EDGE('',*,*,#7243,.F.);
#9551=ORIENTED_EDGE('',*,*,#7230,.F.);
#9552=ORIENTED_EDGE('',*,*,#7247,.F.);
#9553=ORIENTED_EDGE('',*,*,#7196,.T.);
#9554=ORIENTED_EDGE('',*,*,#7248,.T.);
#9555=ORIENTED_EDGE('',*,*,#7246,.T.);
#9556=ORIENTED_EDGE('',*,*,#7233,.F.);
#9557=ORIENTED_EDGE('',*,*,#7249,.T.);
#9558=ORIENTED_EDGE('',*,*,#7250,.T.);
#9559=ORIENTED_EDGE('',*,*,#7251,.T.);
#9560=ORIENTED_EDGE('',*,*,#7197,.T.);
#9561=ORIENTED_EDGE('',*,*,#7247,.T.);
#9562=ORIENTED_EDGE('',*,*,#7232,.F.);
#9563=ORIENTED_EDGE('',*,*,#7241,.F.);
#9564=ORIENTED_EDGE('',*,*,#7252,.F.);
#9565=ORIENTED_EDGE('',*,*,#7249,.F.);
#9566=ORIENTED_EDGE('',*,*,#7253,.T.);
#9567=ORIENTED_EDGE('',*,*,#7240,.F.);
#9568=ORIENTED_EDGE('',*,*,#7254,.T.);
#9569=ORIENTED_EDGE('',*,*,#7255,.T.);
#9570=ORIENTED_EDGE('',*,*,#7256,.T.);
#9571=ORIENTED_EDGE('',*,*,#7250,.F.);
#9572=ORIENTED_EDGE('',*,*,#7252,.T.);
#9573=ORIENTED_EDGE('',*,*,#7257,.T.);
#9574=ORIENTED_EDGE('',*,*,#7244,.T.);
#9575=ORIENTED_EDGE('',*,*,#7248,.F.);
#9576=ORIENTED_EDGE('',*,*,#7195,.T.);
#9577=ORIENTED_EDGE('',*,*,#7258,.T.);
#9578=ORIENTED_EDGE('',*,*,#7257,.F.);
#9579=ORIENTED_EDGE('',*,*,#7194,.T.);
#9580=ORIENTED_EDGE('',*,*,#7259,.T.);
#9581=ORIENTED_EDGE('',*,*,#7260,.T.);
#9582=ORIENTED_EDGE('',*,*,#7261,.T.);
#9583=ORIENTED_EDGE('',*,*,#7210,.T.);
#9584=ORIENTED_EDGE('',*,*,#7238,.F.);
#9585=ORIENTED_EDGE('',*,*,#7262,.T.);
#9586=ORIENTED_EDGE('',*,*,#7263,.T.);
#9587=ORIENTED_EDGE('',*,*,#7261,.F.);
#9588=ORIENTED_EDGE('',*,*,#7264,.T.);
#9589=ORIENTED_EDGE('',*,*,#7262,.F.);
#9590=ORIENTED_EDGE('',*,*,#7265,.T.);
#9591=ORIENTED_EDGE('',*,*,#7266,.T.);
#9592=ORIENTED_EDGE('',*,*,#7267,.T.);
#9593=ORIENTED_EDGE('',*,*,#7268,.T.);
#9594=ORIENTED_EDGE('',*,*,#7269,.T.);
#9595=ORIENTED_EDGE('',*,*,#7266,.F.);
#9596=ORIENTED_EDGE('',*,*,#7270,.T.);
#9597=ORIENTED_EDGE('',*,*,#7193,.T.);
#9598=ORIENTED_EDGE('',*,*,#7268,.F.);
#9599=ORIENTED_EDGE('',*,*,#7271,.T.);
#9600=ORIENTED_EDGE('',*,*,#7259,.F.);
#9601=ORIENTED_EDGE('',*,*,#7239,.F.);
#9602=ORIENTED_EDGE('',*,*,#7245,.F.);
#9603=ORIENTED_EDGE('',*,*,#7258,.F.);
#9604=ORIENTED_EDGE('',*,*,#7272,.T.);
#9605=ORIENTED_EDGE('',*,*,#7273,.T.);
#9606=ORIENTED_EDGE('',*,*,#7271,.F.);
#9607=ORIENTED_EDGE('',*,*,#7270,.F.);
#9608=ORIENTED_EDGE('',*,*,#7265,.F.);
#9609=ORIENTED_EDGE('',*,*,#7264,.F.);
#9610=ORIENTED_EDGE('',*,*,#7260,.F.);
#9611=ORIENTED_EDGE('',*,*,#7272,.F.);
#9612=ORIENTED_EDGE('',*,*,#7274,.T.);
#9613=ORIENTED_EDGE('',*,*,#7275,.T.);
#9614=ORIENTED_EDGE('',*,*,#7276,.T.);
#9615=ORIENTED_EDGE('',*,*,#7191,.T.);
#9616=ORIENTED_EDGE('',*,*,#7277,.T.);
#9617=ORIENTED_EDGE('',*,*,#7190,.T.);
#9618=ORIENTED_EDGE('',*,*,#7278,.T.);
#9619=ORIENTED_EDGE('',*,*,#7223,.T.);
#9620=ORIENTED_EDGE('',*,*,#7277,.F.);
#9621=ORIENTED_EDGE('',*,*,#7279,.T.);
#9622=ORIENTED_EDGE('',*,*,#7280,.T.);
#9623=ORIENTED_EDGE('',*,*,#7276,.F.);
#9624=ORIENTED_EDGE('',*,*,#7281,.T.);
#9625=ORIENTED_EDGE('',*,*,#7282,.T.);
#9626=ORIENTED_EDGE('',*,*,#7283,.T.);
#9627=ORIENTED_EDGE('',*,*,#7279,.F.);
#9628=ORIENTED_EDGE('',*,*,#7284,.T.);
#9629=ORIENTED_EDGE('',*,*,#7285,.T.);
#9630=ORIENTED_EDGE('',*,*,#7286,.T.);
#9631=ORIENTED_EDGE('',*,*,#7282,.F.);
#9632=ORIENTED_EDGE('',*,*,#7287,.T.);
#9633=ORIENTED_EDGE('',*,*,#7212,.T.);
#9634=ORIENTED_EDGE('',*,*,#7285,.F.);
#9635=ORIENTED_EDGE('',*,*,#7288,.T.);
#9636=ORIENTED_EDGE('',*,*,#7219,.F.);
#9637=ORIENTED_EDGE('',*,*,#7288,.F.);
#9638=ORIENTED_EDGE('',*,*,#7287,.F.);
#9639=ORIENTED_EDGE('',*,*,#7284,.F.);
#9640=ORIENTED_EDGE('',*,*,#7281,.F.);
#9641=ORIENTED_EDGE('',*,*,#7275,.F.);
#9642=ORIENTED_EDGE('',*,*,#7222,.T.);
#9643=ORIENTED_EDGE('',*,*,#7289,.T.);
#9644=ORIENTED_EDGE('',*,*,#7290,.T.);
#9645=ORIENTED_EDGE('',*,*,#7188,.T.);
#9646=ORIENTED_EDGE('',*,*,#7127,.F.);
#9647=ORIENTED_EDGE('',*,*,#7151,.T.);
#9648=ORIENTED_EDGE('',*,*,#7169,.F.);
#9649=ORIENTED_EDGE('',*,*,#7199,.T.);
#9650=ORIENTED_EDGE('',*,*,#7291,.T.);
#9651=ORIENTED_EDGE('',*,*,#7292,.T.);
#9652=ORIENTED_EDGE('',*,*,#7293,.T.);
#9653=ORIENTED_EDGE('',*,*,#7294,.T.);
#9654=ORIENTED_EDGE('',*,*,#7166,.F.);
#9655=ORIENTED_EDGE('',*,*,#7294,.F.);
#9656=ORIENTED_EDGE('',*,*,#7295,.T.);
#9657=ORIENTED_EDGE('',*,*,#7215,.T.);
#9658=ORIENTED_EDGE('',*,*,#7187,.F.);
#9659=ORIENTED_EDGE('',*,*,#7296,.T.);
#9660=ORIENTED_EDGE('',*,*,#7251,.F.);
#9661=ORIENTED_EDGE('',*,*,#7256,.F.);
#9662=ORIENTED_EDGE('',*,*,#7297,.T.);
#9663=ORIENTED_EDGE('',*,*,#7298,.F.);
#9664=ORIENTED_EDGE('',*,*,#7291,.F.);
#9665=ORIENTED_EDGE('',*,*,#7198,.T.);
#9666=ORIENTED_EDGE('',*,*,#7167,.F.);
#9667=ORIENTED_EDGE('',*,*,#7296,.F.);
#9668=ORIENTED_EDGE('',*,*,#7186,.F.);
#9669=ORIENTED_EDGE('',*,*,#7299,.F.);
#9670=ORIENTED_EDGE('',*,*,#7242,.F.);
#9671=ORIENTED_EDGE('',*,*,#7205,.T.);
#9672=ORIENTED_EDGE('',*,*,#7218,.F.);
#9673=ORIENTED_EDGE('',*,*,#7300,.F.);
#9674=ORIENTED_EDGE('',*,*,#7301,.T.);
#9675=ORIENTED_EDGE('',*,*,#7254,.F.);
#9676=ORIENTED_EDGE('',*,*,#7255,.F.);
#9677=ORIENTED_EDGE('',*,*,#7301,.F.);
#9678=ORIENTED_EDGE('',*,*,#7302,.F.);
#9679=ORIENTED_EDGE('',*,*,#7297,.F.);
#9680=ORIENTED_EDGE('',*,*,#7303,.F.);
#9681=ORIENTED_EDGE('',*,*,#7304,.F.);
#9682=ORIENTED_EDGE('',*,*,#7305,.F.);
#9683=ORIENTED_EDGE('',*,*,#7306,.F.);
#9684=ORIENTED_EDGE('',*,*,#7292,.F.);
#9685=ORIENTED_EDGE('',*,*,#7298,.T.);
#9686=ORIENTED_EDGE('',*,*,#7302,.T.);
#9687=ORIENTED_EDGE('',*,*,#7300,.T.);
#9688=ORIENTED_EDGE('',*,*,#7217,.F.);
#9689=ORIENTED_EDGE('',*,*,#7307,.T.);
#9690=ORIENTED_EDGE('',*,*,#7305,.T.);
#9691=ORIENTED_EDGE('',*,*,#7308,.T.);
#9692=ORIENTED_EDGE('',*,*,#7309,.T.);
#9693=ORIENTED_EDGE('',*,*,#7310,.T.);
#9694=ORIENTED_EDGE('',*,*,#7303,.T.);
#9695=ORIENTED_EDGE('',*,*,#7311,.T.);
#9696=ORIENTED_EDGE('',*,*,#7312,.T.);
#9697=ORIENTED_EDGE('',*,*,#7313,.T.);
#9698=ORIENTED_EDGE('',*,*,#7314,.T.);
#9699=ORIENTED_EDGE('',*,*,#7315,.T.);
#9700=ORIENTED_EDGE('',*,*,#7311,.F.);
#9701=ORIENTED_EDGE('',*,*,#7306,.T.);
#9702=ORIENTED_EDGE('',*,*,#7310,.F.);
#9703=ORIENTED_EDGE('',*,*,#7316,.T.);
#9704=ORIENTED_EDGE('',*,*,#7304,.T.);
#9705=ORIENTED_EDGE('',*,*,#7313,.F.);
#9706=ORIENTED_EDGE('',*,*,#7317,.T.);
#9707=ORIENTED_EDGE('',*,*,#7318,.T.);
#9708=ORIENTED_EDGE('',*,*,#7319,.T.);
#9709=ORIENTED_EDGE('',*,*,#7308,.F.);
#9710=ORIENTED_EDGE('',*,*,#7318,.F.);
#9711=ORIENTED_EDGE('',*,*,#7320,.F.);
#9712=ORIENTED_EDGE('',*,*,#7321,.F.);
#9713=ORIENTED_EDGE('',*,*,#7322,.F.);
#9714=ORIENTED_EDGE('',*,*,#7323,.F.);
#9715=ORIENTED_EDGE('',*,*,#7324,.F.);
#9716=ORIENTED_EDGE('',*,*,#7312,.F.);
#9717=ORIENTED_EDGE('',*,*,#7315,.F.);
#9718=ORIENTED_EDGE('',*,*,#7325,.T.);
#9719=ORIENTED_EDGE('',*,*,#7326,.F.);
#9720=ORIENTED_EDGE('',*,*,#7320,.T.);
#9721=ORIENTED_EDGE('',*,*,#7317,.F.);
#9722=ORIENTED_EDGE('',*,*,#7327,.T.);
#9723=ORIENTED_EDGE('',*,*,#7328,.T.);
#9724=ORIENTED_EDGE('',*,*,#7329,.T.);
#9725=ORIENTED_EDGE('',*,*,#7330,.T.);
#9726=ORIENTED_EDGE('',*,*,#7331,.T.);
#9727=ORIENTED_EDGE('',*,*,#7332,.T.);
#9728=ORIENTED_EDGE('',*,*,#7333,.T.);
#9729=ORIENTED_EDGE('',*,*,#7334,.T.);
#9730=ORIENTED_EDGE('',*,*,#7322,.T.);
#9731=ORIENTED_EDGE('',*,*,#7335,.T.);
#9732=ORIENTED_EDGE('',*,*,#7332,.F.);
#9733=ORIENTED_EDGE('',*,*,#7336,.T.);
#9734=ORIENTED_EDGE('',*,*,#7330,.F.);
#9735=ORIENTED_EDGE('',*,*,#7337,.T.);
#9736=ORIENTED_EDGE('',*,*,#7338,.T.);
#9737=ORIENTED_EDGE('',*,*,#7334,.F.);
#9738=ORIENTED_EDGE('',*,*,#7339,.T.);
#9739=ORIENTED_EDGE('',*,*,#7340,.T.);
#9740=ORIENTED_EDGE('',*,*,#7341,.T.);
#9741=ORIENTED_EDGE('',*,*,#7328,.F.);
#9742=ORIENTED_EDGE('',*,*,#7314,.F.);
#9743=ORIENTED_EDGE('',*,*,#7342,.F.);
#9744=ORIENTED_EDGE('',*,*,#7343,.F.);
#9745=ORIENTED_EDGE('',*,*,#7340,.F.);
#9746=ORIENTED_EDGE('',*,*,#7344,.F.);
#9747=ORIENTED_EDGE('',*,*,#7325,.F.);
#9748=ORIENTED_EDGE('',*,*,#7333,.F.);
#9749=ORIENTED_EDGE('',*,*,#7335,.F.);
#9750=ORIENTED_EDGE('',*,*,#7321,.T.);
#9751=ORIENTED_EDGE('',*,*,#7326,.T.);
#9752=ORIENTED_EDGE('',*,*,#7344,.T.);
#9753=ORIENTED_EDGE('',*,*,#7339,.F.);
#9754=ORIENTED_EDGE('',*,*,#7345,.F.);
#9755=ORIENTED_EDGE('',*,*,#7225,.F.);
#9756=ORIENTED_EDGE('',*,*,#7346,.F.);
#9757=ORIENTED_EDGE('',*,*,#7149,.T.);
#9758=ORIENTED_EDGE('',*,*,#7331,.F.);
#9759=ORIENTED_EDGE('',*,*,#7338,.F.);
#9760=ORIENTED_EDGE('',*,*,#7327,.F.);
#9761=ORIENTED_EDGE('',*,*,#7336,.F.);
#9762=ORIENTED_EDGE('',*,*,#7226,.T.);
#9763=ORIENTED_EDGE('',*,*,#7345,.T.);
#9764=ORIENTED_EDGE('',*,*,#7148,.T.);
#9765=ORIENTED_EDGE('',*,*,#7144,.F.);
#9766=ORIENTED_EDGE('',*,*,#7214,.T.);
#9767=ORIENTED_EDGE('',*,*,#7221,.F.);
#9768=ORIENTED_EDGE('',*,*,#7293,.F.);
#9769=ORIENTED_EDGE('',*,*,#7307,.F.);
#9770=ORIENTED_EDGE('',*,*,#7216,.F.);
#9771=ORIENTED_EDGE('',*,*,#7295,.F.);
#9772=ORIENTED_EDGE('',*,*,#7347,.T.);
#9773=ORIENTED_EDGE('',*,*,#7224,.T.);
#9774=ORIENTED_EDGE('',*,*,#7278,.F.);
#9775=ORIENTED_EDGE('',*,*,#7189,.T.);
#9776=ORIENTED_EDGE('',*,*,#7290,.F.);
#9777=ORIENTED_EDGE('',*,*,#7150,.T.);
#9778=ORIENTED_EDGE('',*,*,#7346,.T.);
#9779=ORIENTED_EDGE('',*,*,#7329,.F.);
#9780=ORIENTED_EDGE('',*,*,#7341,.F.);
#9781=ORIENTED_EDGE('',*,*,#7343,.T.);
#9782=ORIENTED_EDGE('',*,*,#7348,.F.);
#9783=ORIENTED_EDGE('',*,*,#7323,.T.);
#9784=ORIENTED_EDGE('',*,*,#7337,.F.);
#9785=ORIENTED_EDGE('',*,*,#7309,.F.);
#9786=ORIENTED_EDGE('',*,*,#7319,.F.);
#9787=ORIENTED_EDGE('',*,*,#7324,.T.);
#9788=ORIENTED_EDGE('',*,*,#7348,.T.);
#9789=ORIENTED_EDGE('',*,*,#7342,.T.);
#9790=ORIENTED_EDGE('',*,*,#7316,.F.);
#9791=ORIENTED_EDGE('',*,*,#7253,.F.);
#9792=ORIENTED_EDGE('',*,*,#7349,.T.);
#9793=ORIENTED_EDGE('',*,*,#7273,.F.);
#9794=ORIENTED_EDGE('',*,*,#7349,.F.);
#9795=ORIENTED_EDGE('',*,*,#7347,.F.);
#9796=ORIENTED_EDGE('',*,*,#7350,.T.);
#9797=ORIENTED_EDGE('',*,*,#7351,.F.);
#9798=ORIENTED_EDGE('',*,*,#7350,.F.);
#9799=ORIENTED_EDGE('',*,*,#7352,.F.);
#9800=ORIENTED_EDGE('',*,*,#7353,.T.);
#9801=ORIENTED_EDGE('',*,*,#7147,.F.);
#9802=ORIENTED_EDGE('',*,*,#7353,.F.);
#9803=ORIENTED_EDGE('',*,*,#7274,.F.);
#9804=ORIENTED_EDGE('',*,*,#7354,.T.);
#9805=ORIENTED_EDGE('',*,*,#7289,.F.);
#9806=ORIENTED_EDGE('',*,*,#7354,.F.);
#9807=ORIENTED_EDGE('',*,*,#7269,.F.);
#9808=ORIENTED_EDGE('',*,*,#7192,.T.);
#9809=ORIENTED_EDGE('',*,*,#7280,.F.);
#9810=ORIENTED_EDGE('',*,*,#7355,.T.);
#9811=ORIENTED_EDGE('',*,*,#7263,.F.);
#9812=ORIENTED_EDGE('',*,*,#7356,.T.);
#9813=ORIENTED_EDGE('',*,*,#7286,.F.);
#9814=ORIENTED_EDGE('',*,*,#7211,.T.);
#9815=ORIENTED_EDGE('',*,*,#7164,.F.);
#9816=ORIENTED_EDGE('',*,*,#7299,.T.);
#9817=ORIENTED_EDGE('',*,*,#7181,.F.);
#9818=ORIENTED_EDGE('',*,*,#7357,.T.);
#9819=ORIENTED_EDGE('',*,*,#7162,.F.);
#9820=ORIENTED_EDGE('',*,*,#7357,.F.);
#9821=ORIENTED_EDGE('',*,*,#7152,.F.);
#9822=ORIENTED_EDGE('',*,*,#7358,.F.);
#9823=ORIENTED_EDGE('',*,*,#7351,.T.);
#9824=ORIENTED_EDGE('',*,*,#7267,.F.);
#9825=ORIENTED_EDGE('',*,*,#7355,.F.);
#9826=ORIENTED_EDGE('',*,*,#7283,.F.);
#9827=ORIENTED_EDGE('',*,*,#7356,.F.);
#9828=ORIENTED_EDGE('',*,*,#7156,.F.);
#9829=ORIENTED_EDGE('',*,*,#7358,.T.);
#9830=ORIENTED_EDGE('',*,*,#7180,.F.);
#9831=ORIENTED_EDGE('',*,*,#7178,.F.);
#9832=ORIENTED_EDGE('',*,*,#7175,.F.);
#9833=ORIENTED_EDGE('',*,*,#7172,.F.);
#9834=ORIENTED_EDGE('',*,*,#7352,.T.);
#13487=PLANE('',#14998);
#13488=PLANE('',#15002);
#13489=PLANE('',#15006);
#13490=PLANE('',#15007);
#13491=PLANE('',#15008);
#13492=PLANE('',#15010);
#13493=PLANE('',#15011);
#13494=PLANE('',#15012);
#13495=PLANE('',#15013);
#13496=PLANE('',#15017);
#13497=PLANE('',#15021);
#13498=PLANE('',#15025);
#13499=PLANE('',#15029);
#13500=PLANE('',#15030);
#13501=PLANE('',#15035);
#13502=PLANE('',#15037);
#13503=PLANE('',#15041);
#13504=PLANE('',#15042);
#13505=PLANE('',#15043);
#13506=PLANE('',#15044);
#13507=PLANE('',#15045);
#13508=PLANE('',#15046);
#13509=PLANE('',#15049);
#13510=PLANE('',#15050);
#13511=PLANE('',#15053);
#13512=PLANE('',#15054);
#13513=PLANE('',#15055);
#13514=PLANE('',#15056);
#13515=PLANE('',#15058);
#13516=PLANE('',#15060);
#13517=PLANE('',#15061);
#13518=PLANE('',#15065);
#13519=PLANE('',#15069);
#13520=PLANE('',#15070);
#13521=PLANE('',#15072);
#13522=PLANE('',#15074);
#13523=PLANE('',#15075);
#13524=PLANE('',#15079);
#13525=PLANE('',#15083);
#13526=PLANE('',#15084);
#13527=PLANE('',#15086);
#13528=PLANE('',#15087);
#13529=PLANE('',#15088);
#13530=PLANE('',#15091);
#13531=PLANE('',#15097);
#13532=PLANE('',#15098);
#13533=PLANE('',#15099);
#13534=PLANE('',#15104);
#13535=PLANE('',#15106);
#13536=PLANE('',#15107);
#13537=PLANE('',#15108);
#13538=PLANE('',#15114);
#13539=PLANE('',#15115);
#13540=PLANE('',#15120);
#13541=PLANE('',#15123);
#13542=PLANE('',#15124);
#13543=PLANE('',#15134);
#13544=PLANE('',#15135);
#13545=PLANE('',#15136);
#13978=ADVANCED_FACE('',(#1410),#13487,.T.);
#13979=ADVANCED_FACE('',(#1411),#1291,.T.);
#13980=ADVANCED_FACE('',(#1412),#13488,.T.);
#13981=ADVANCED_FACE('',(#1413),#1292,.T.);
#13982=ADVANCED_FACE('',(#1414),#13489,.T.);
#13983=ADVANCED_FACE('',(#1415),#13490,.T.);
#13984=ADVANCED_FACE('',(#1416,#644),#13491,.T.);
#13985=ADVANCED_FACE('',(#1417),#13492,.T.);
#13986=ADVANCED_FACE('',(#1418),#13493,.T.);
#13987=ADVANCED_FACE('',(#1419),#13494,.T.);
#13988=ADVANCED_FACE('',(#1420),#13495,.T.);
#13989=ADVANCED_FACE('',(#1421),#1293,.T.);
#13990=ADVANCED_FACE('',(#1422),#13496,.T.);
#13991=ADVANCED_FACE('',(#1423),#1294,.T.);
#13992=ADVANCED_FACE('',(#1424),#13497,.T.);
#13993=ADVANCED_FACE('',(#1425),#1295,.T.);
#13994=ADVANCED_FACE('',(#1426),#13498,.T.);
#13995=ADVANCED_FACE('',(#1427),#1296,.T.);
#13996=ADVANCED_FACE('',(#1428),#13499,.T.);
#13997=ADVANCED_FACE('',(#1429),#13500,.F.);
#13998=ADVANCED_FACE('',(#1430),#696,.T.);
#13999=ADVANCED_FACE('',(#1431),#13501,.T.);
#14000=ADVANCED_FACE('',(#1432),#697,.T.);
#14001=ADVANCED_FACE('',(#1433),#13502,.T.);
#14002=ADVANCED_FACE('',(#1434),#13503,.T.);
#14003=ADVANCED_FACE('',(#1435),#13504,.T.);
#14004=ADVANCED_FACE('',(#1436),#13505,.T.);
#14005=ADVANCED_FACE('',(#1437),#13506,.T.);
#14006=ADVANCED_FACE('',(#1438),#13507,.T.);
#14007=ADVANCED_FACE('',(#1439),#13508,.T.);
#14008=ADVANCED_FACE('',(#1440),#1297,.T.);
#14009=ADVANCED_FACE('',(#1441),#13509,.T.);
#14010=ADVANCED_FACE('',(#1442),#13510,.T.);
#14011=ADVANCED_FACE('',(#1443),#698,.T.);
#14012=ADVANCED_FACE('',(#1444),#13511,.T.);
#14013=ADVANCED_FACE('',(#1445),#13512,.T.);
#14014=ADVANCED_FACE('',(#1446),#13513,.T.);
#14015=ADVANCED_FACE('',(#1447,#645),#13514,.T.);
#14016=ADVANCED_FACE('',(#1448),#13515,.T.);
#14017=ADVANCED_FACE('',(#1449),#1298,.T.);
#14018=ADVANCED_FACE('',(#1450),#13516,.T.);
#14019=ADVANCED_FACE('',(#1451),#13517,.T.);
#14020=ADVANCED_FACE('',(#1452),#1299,.T.);
#14021=ADVANCED_FACE('',(#1453),#13518,.T.);
#14022=ADVANCED_FACE('',(#1454),#1300,.T.);
#14023=ADVANCED_FACE('',(#1455),#13519,.T.);
#14024=ADVANCED_FACE('',(#1456,#646),#13520,.T.);
#14025=ADVANCED_FACE('',(#1457,#647),#13521,.T.);
#14026=ADVANCED_FACE('',(#1458),#13522,.T.);
#14027=ADVANCED_FACE('',(#1459),#13523,.T.);
#14028=ADVANCED_FACE('',(#1460),#1301,.T.);
#14029=ADVANCED_FACE('',(#1461),#13524,.T.);
#14030=ADVANCED_FACE('',(#1462),#1302,.T.);
#14031=ADVANCED_FACE('',(#1463),#13525,.T.);
#14032=ADVANCED_FACE('',(#1464,#648),#13526,.T.);
#14033=ADVANCED_FACE('',(#1465),#13527,.T.);
#14034=ADVANCED_FACE('',(#1466),#13528,.T.);
#14035=ADVANCED_FACE('',(#1467),#13529,.T.);
#14036=ADVANCED_FACE('',(#1468),#1303,.F.);
#14037=ADVANCED_FACE('',(#1469),#13530,.T.);
#14038=ADVANCED_FACE('',(#1470),#1304,.F.);
#14039=ADVANCED_FACE('',(#1471,#649),#699,.F.);
#14040=ADVANCED_FACE('',(#1472),#13531,.T.);
#14041=ADVANCED_FACE('',(#1473),#13532,.T.);
#14042=ADVANCED_FACE('',(#1474),#13533,.T.);
#14043=ADVANCED_FACE('',(#1475),#1305,.F.);
#14044=ADVANCED_FACE('',(#1476),#1306,.F.);
#14045=ADVANCED_FACE('',(#1477),#13534,.T.);
#14046=ADVANCED_FACE('',(#1478),#13535,.F.);
#14047=ADVANCED_FACE('',(#1479),#13536,.T.);
#14048=ADVANCED_FACE('',(#1480),#13537,.T.);
#14049=ADVANCED_FACE('',(#1481),#1307,.T.);
#14050=ADVANCED_FACE('',(#1482),#1308,.T.);
#14051=ADVANCED_FACE('',(#1483),#13538,.F.);
#14052=ADVANCED_FACE('',(#1484),#13539,.F.);
#14053=ADVANCED_FACE('',(#1485,#650),#700,.T.);
#14054=ADVANCED_FACE('',(#1486),#1309,.T.);
#14055=ADVANCED_FACE('',(#1487,#651),#13540,.T.);
#14056=ADVANCED_FACE('',(#1488),#1310,.T.);
#14057=ADVANCED_FACE('',(#1489),#13541,.F.);
#14058=ADVANCED_FACE('',(#1490),#13542,.F.);
#14059=ADVANCED_FACE('',(#1491),#701,.F.);
#14060=ADVANCED_FACE('',(#1492),#702,.F.);
#14061=ADVANCED_FACE('',(#1493),#703,.F.);
#14062=ADVANCED_FACE('',(#1494),#704,.F.);
#14063=ADVANCED_FACE('',(#1495),#705,.T.);
#14064=ADVANCED_FACE('',(#1496),#706,.T.);
#14065=ADVANCED_FACE('',(#1497),#707,.T.);
#14066=ADVANCED_FACE('',(#1498,#652),#13543,.T.);
#14067=ADVANCED_FACE('',(#1499),#13544,.T.);
#14068=ADVANCED_FACE('',(#1500,#653),#13545,.T.);
#14777=CLOSED_SHELL('',(#13978,#13979,#13980,#13981,#13982,#13983,#13984,
#13985,#13986,#13987,#13988,#13989,#13990,#13991,#13992,#13993,#13994,#13995,
#13996,#13997,#13998,#13999,#14000,#14001,#14002,#14003,#14004,#14005,#14006,
#14007,#14008,#14009,#14010,#14011,#14012,#14013,#14014,#14015,#14016,#14017,
#14018,#14019,#14020,#14021,#14022,#14023,#14024,#14025,#14026,#14027,#14028,
#14029,#14030,#14031,#14032,#14033,#14034,#14035,#14036,#14037,#14038,#14039,
#14040,#14041,#14042,#14043,#14044,#14045,#14046,#14047,#14048,#14049,#14050,
#14051,#14052,#14053,#14054,#14055,#14056,#14057,#14058,#14059,#14060,#14061,
#14062,#14063,#14064,#14065,#14066,#14067,#14068));
#14997=AXIS2_PLACEMENT_3D('',#19984,#16317,#16318);
#14998=AXIS2_PLACEMENT_3D('',#19985,#16319,#16320);
#14999=AXIS2_PLACEMENT_3D('',#19994,#16325,#16326);
#15000=AXIS2_PLACEMENT_3D('',#19996,#16327,#16328);
#15001=AXIS2_PLACEMENT_3D('',#19999,#16330,#16331);
#15002=AXIS2_PLACEMENT_3D('',#20000,#16332,#16333);
#15003=AXIS2_PLACEMENT_3D('',#20006,#16337,#16338);
#15004=AXIS2_PLACEMENT_3D('',#20008,#16339,#16340);
#15005=AXIS2_PLACEMENT_3D('',#20011,#16342,#16343);
#15006=AXIS2_PLACEMENT_3D('',#20012,#16344,#16345);
#15007=AXIS2_PLACEMENT_3D('',#20018,#16349,#16350);
#15008=AXIS2_PLACEMENT_3D('',#20026,#16353,#16354);
#15009=AXIS2_PLACEMENT_3D('',#20029,#16356,#16357);
#15010=AXIS2_PLACEMENT_3D('',#20030,#16358,#16359);
#15011=AXIS2_PLACEMENT_3D('',#20042,#16362,#16363);
#15012=AXIS2_PLACEMENT_3D('',#20051,#16368,#16369);
#15013=AXIS2_PLACEMENT_3D('',#20060,#16374,#16375);
#15014=AXIS2_PLACEMENT_3D('',#20066,#16379,#16380);
#15015=AXIS2_PLACEMENT_3D('',#20070,#16382,#16383);
#15016=AXIS2_PLACEMENT_3D('',#20071,#16384,#16385);
#15017=AXIS2_PLACEMENT_3D('',#20072,#16386,#16387);
#15018=AXIS2_PLACEMENT_3D('',#20080,#16392,#16393);
#15019=AXIS2_PLACEMENT_3D('',#20084,#16395,#16396);
#15020=AXIS2_PLACEMENT_3D('',#20085,#16397,#16398);
#15021=AXIS2_PLACEMENT_3D('',#20086,#16399,#16400);
#15022=AXIS2_PLACEMENT_3D('',#20092,#16404,#16405);
#15023=AXIS2_PLACEMENT_3D('',#20096,#16407,#16408);
#15024=AXIS2_PLACEMENT_3D('',#20097,#16409,#16410);
#15025=AXIS2_PLACEMENT_3D('',#20098,#16411,#16412);
#15026=AXIS2_PLACEMENT_3D('',#20101,#16415,#16416);
#15027=AXIS2_PLACEMENT_3D('',#20103,#16417,#16418);
#15028=AXIS2_PLACEMENT_3D('',#20106,#16420,#16421);
#15029=AXIS2_PLACEMENT_3D('',#20107,#16422,#16423);
#15030=AXIS2_PLACEMENT_3D('',#20115,#16428,#16429);
#15031=AXIS2_PLACEMENT_3D('',#20119,#16431,#16432);
#15032=AXIS2_PLACEMENT_3D('',#20131,#16438,#16439);
#15033=AXIS2_PLACEMENT_3D('',#20137,#16442,#16443);
#15034=AXIS2_PLACEMENT_3D('',#20140,#16446,#16447);
#15035=AXIS2_PLACEMENT_3D('',#20142,#16449,#16450);
#15036=AXIS2_PLACEMENT_3D('',#20144,#16452,#16453);
#15037=AXIS2_PLACEMENT_3D('',#20146,#16455,#16456);
#15038=AXIS2_PLACEMENT_3D('',#20150,#16458,#16459);
#15039=AXIS2_PLACEMENT_3D('',#20156,#16462,#16463);
#15040=AXIS2_PLACEMENT_3D('',#20167,#16469,#16470);
#15041=AXIS2_PLACEMENT_3D('',#20168,#16471,#16472);
#15042=AXIS2_PLACEMENT_3D('',#20178,#16476,#16477);
#15043=AXIS2_PLACEMENT_3D('',#20186,#16480,#16481);
#15044=AXIS2_PLACEMENT_3D('',#20200,#16485,#16486);
#15045=AXIS2_PLACEMENT_3D('',#20206,#16490,#16491);
#15046=AXIS2_PLACEMENT_3D('',#20214,#16496,#16497);
#15047=AXIS2_PLACEMENT_3D('',#20218,#16500,#16501);
#15048=AXIS2_PLACEMENT_3D('',#20220,#16502,#16503);
#15049=AXIS2_PLACEMENT_3D('',#20222,#16505,#16506);
#15050=AXIS2_PLACEMENT_3D('',#20226,#16509,#16510);
#15051=AXIS2_PLACEMENT_3D('',#20234,#16513,#16514);
#15052=AXIS2_PLACEMENT_3D('',#20238,#16516,#16517);
#15053=AXIS2_PLACEMENT_3D('',#20240,#16519,#16520);
#15054=AXIS2_PLACEMENT_3D('',#20242,#16522,#16523);
#15055=AXIS2_PLACEMENT_3D('',#20245,#16526,#16527);
#15056=AXIS2_PLACEMENT_3D('',#20253,#16530,#16531);
#15057=AXIS2_PLACEMENT_3D('',#20256,#16533,#16534);
#15058=AXIS2_PLACEMENT_3D('',#20257,#16535,#16536);
#15059=AXIS2_PLACEMENT_3D('',#20267,#16538,#16539);
#15060=AXIS2_PLACEMENT_3D('',#20269,#16541,#16542);
#15061=AXIS2_PLACEMENT_3D('',#20273,#16545,#16546);
#15062=AXIS2_PLACEMENT_3D('',#20277,#16549,#16550);
#15063=AXIS2_PLACEMENT_3D('',#20281,#16552,#16553);
#15064=AXIS2_PLACEMENT_3D('',#20282,#16554,#16555);
#15065=AXIS2_PLACEMENT_3D('',#20283,#16556,#16557);
#15066=AXIS2_PLACEMENT_3D('',#20289,#16561,#16562);
#15067=AXIS2_PLACEMENT_3D('',#20292,#16564,#16565);
#15068=AXIS2_PLACEMENT_3D('',#20293,#16566,#16567);
#15069=AXIS2_PLACEMENT_3D('',#20294,#16568,#16569);
#15070=AXIS2_PLACEMENT_3D('',#20296,#16571,#16572);
#15071=AXIS2_PLACEMENT_3D('',#20299,#16574,#16575);
#15072=AXIS2_PLACEMENT_3D('',#20300,#16576,#16577);
#15073=AXIS2_PLACEMENT_3D('',#20302,#16578,#16579);
#15074=AXIS2_PLACEMENT_3D('',#20303,#16580,#16581);
#15075=AXIS2_PLACEMENT_3D('',#20308,#16585,#16586);
#15076=AXIS2_PLACEMENT_3D('',#20312,#16587,#16588);
#15077=AXIS2_PLACEMENT_3D('',#20316,#16590,#16591);
#15078=AXIS2_PLACEMENT_3D('',#20317,#16592,#16593);
#15079=AXIS2_PLACEMENT_3D('',#20318,#16594,#16595);
#15080=AXIS2_PLACEMENT_3D('',#20324,#16599,#16600);
#15081=AXIS2_PLACEMENT_3D('',#20327,#16602,#16603);
#15082=AXIS2_PLACEMENT_3D('',#20328,#16604,#16605);
#15083=AXIS2_PLACEMENT_3D('',#20329,#16606,#16607);
#15084=AXIS2_PLACEMENT_3D('',#20331,#16609,#16610);
#15085=AXIS2_PLACEMENT_3D('',#20333,#16611,#16612);
#15086=AXIS2_PLACEMENT_3D('',#20334,#16613,#16614);
#15087=AXIS2_PLACEMENT_3D('',#20338,#16615,#16616);
#15088=AXIS2_PLACEMENT_3D('',#20348,#16620,#16621);
#15089=AXIS2_PLACEMENT_3D('',#20351,#16624,#16625);
#15090=AXIS2_PLACEMENT_3D('',#20353,#16626,#16627);
#15091=AXIS2_PLACEMENT_3D('',#20357,#16628,#16629);
#15092=AXIS2_PLACEMENT_3D('',#20359,#16631,#16632);
#15093=AXIS2_PLACEMENT_3D('',#20364,#16633,#16634);
#15094=AXIS2_PLACEMENT_3D('',#20365,#16635,#16636);
#15095=AXIS2_PLACEMENT_3D('',#20371,#16639,#16640);
#15096=AXIS2_PLACEMENT_3D('',#20374,#16642,#16643);
#15097=AXIS2_PLACEMENT_3D('',#20375,#16644,#16645);
#15098=AXIS2_PLACEMENT_3D('',#20377,#16647,#16648);
#15099=AXIS2_PLACEMENT_3D('',#20389,#16650,#16651);
#15100=AXIS2_PLACEMENT_3D('',#20401,#16653,#16654);
#15101=AXIS2_PLACEMENT_3D('',#20404,#16655,#16656);
#15102=AXIS2_PLACEMENT_3D('',#20411,#16657,#16658);
#15103=AXIS2_PLACEMENT_3D('',#20417,#16659,#16660);
#15104=AXIS2_PLACEMENT_3D('',#20421,#16661,#16662);
#15105=AXIS2_PLACEMENT_3D('',#20427,#16665,#16666);
#15106=AXIS2_PLACEMENT_3D('',#20431,#16669,#16670);
#15107=AXIS2_PLACEMENT_3D('',#20435,#16673,#16674);
#15108=AXIS2_PLACEMENT_3D('',#20450,#16677,#16678);
#15109=AXIS2_PLACEMENT_3D('',#20465,#16681,#16682);
#15110=AXIS2_PLACEMENT_3D('',#20469,#16683,#16684);
#15111=AXIS2_PLACEMENT_3D('',#20473,#16685,#16686);
#15112=AXIS2_PLACEMENT_3D('',#20474,#16687,#16688);
#15113=AXIS2_PLACEMENT_3D('',#20480,#16689,#16690);
#15114=AXIS2_PLACEMENT_3D('',#20484,#16691,#16692);
#15115=AXIS2_PLACEMENT_3D('',#20489,#16696,#16697);
#15116=AXIS2_PLACEMENT_3D('',#20490,#16698,#16699);
#15117=AXIS2_PLACEMENT_3D('',#20491,#16700,#16701);
#15118=AXIS2_PLACEMENT_3D('',#20492,#16702,#16703);
#15119=AXIS2_PLACEMENT_3D('',#20493,#16704,#16705);
#15120=AXIS2_PLACEMENT_3D('',#20494,#16706,#16707);
#15121=AXIS2_PLACEMENT_3D('',#20496,#16708,#16709);
#15122=AXIS2_PLACEMENT_3D('',#20497,#16710,#16711);
#15123=AXIS2_PLACEMENT_3D('',#20498,#16712,#16713);
#15124=AXIS2_PLACEMENT_3D('',#20500,#16715,#16716);
#15125=AXIS2_PLACEMENT_3D('',#20501,#16717,#16718);
#15126=AXIS2_PLACEMENT_3D('',#20503,#16720,#16721);
#15127=AXIS2_PLACEMENT_3D('',#20506,#16723,#16724);
#15128=AXIS2_PLACEMENT_3D('',#20507,#16725,#16726);
#15129=AXIS2_PLACEMENT_3D('',#20509,#16727,#16728);
#15130=AXIS2_PLACEMENT_3D('',#20511,#16730,#16731);
#15131=AXIS2_PLACEMENT_3D('',#20513,#16733,#16734);
#15132=AXIS2_PLACEMENT_3D('',#20515,#16736,#16737);
#15133=AXIS2_PLACEMENT_3D('',#20517,#16739,#16740);
#15134=AXIS2_PLACEMENT_3D('',#20519,#16742,#16743);
#15135=AXIS2_PLACEMENT_3D('',#20521,#16745,#16746);
#15136=AXIS2_PLACEMENT_3D('',#20522,#16747,#16748);
#16317=DIRECTION('axis',(0.,0.,1.));
#16318=DIRECTION('refdir',(1.,0.,0.));
#16319=DIRECTION('center_axis',(0.707106781186548,-0.707106781186548,0.));
#16320=DIRECTION('ref_axis',(0.,0.,-1.));
#16321=DIRECTION('',(0.577350269189626,0.577350269189626,-0.577350269189626));
#16322=DIRECTION('',(0.,0.,-1.));
#16323=DIRECTION('',(0.707106781186547,0.707106781186547,0.));
#16324=DIRECTION('',(0.,0.,1.));
#16325=DIRECTION('center_axis',(-1.,0.,0.));
#16326=DIRECTION('ref_axis',(0.,-0.707106781186547,-0.707106781186548));
#16327=DIRECTION('center_axis',(1.,0.,0.));
#16328=DIRECTION('ref_axis',(0.,-0.707106781186547,-0.707106781186548));
#16329=DIRECTION('',(0.707106781186551,4.08878244448901E-16,0.707106781186544));
#16330=DIRECTION('center_axis',(-1.,0.,0.));
#16331=DIRECTION('ref_axis',(0.,-0.707106781186547,-0.707106781186548));
#16332=DIRECTION('center_axis',(0.707106781186548,0.,-0.707106781186548));
#16333=DIRECTION('ref_axis',(-0.707106781186548,0.,-0.707106781186548));
#16334=DIRECTION('',(0.707106781186547,0.,0.707106781186547));
#16335=DIRECTION('',(0.,-1.,0.));
#16336=DIRECTION('',(0.,1.,0.));
#16337=DIRECTION('center_axis',(-1.,0.,0.));
#16338=DIRECTION('ref_axis',(0.,0.707106781186547,-0.707106781186548));
#16339=DIRECTION('center_axis',(1.,0.,0.));
#16340=DIRECTION('ref_axis',(0.,0.707106781186547,-0.707106781186548));
#16341=DIRECTION('',(0.707106781186549,-0.707106781186546,0.));
#16342=DIRECTION('center_axis',(-1.,0.,0.));
#16343=DIRECTION('ref_axis',(0.,0.707106781186547,-0.707106781186548));
#16344=DIRECTION('center_axis',(0.707106781186548,0.707106781186548,0.));
#16345=DIRECTION('ref_axis',(0.,0.,-1.));
#16346=DIRECTION('',(0.,0.,-1.));
#16347=DIRECTION('',(0.,0.,1.));
#16348=DIRECTION('',(0.577350269189626,-0.577350269189626,-0.577350269189626));
#16349=DIRECTION('center_axis',(0.,0.707106781186548,-0.707106781186548));
#16350=DIRECTION('ref_axis',(-1.,0.,0.));
#16351=DIRECTION('',(1.,0.,0.));
#16352=DIRECTION('',(-1.,0.,0.));
#16353=DIRECTION('center_axis',(1.,0.,0.));
#16354=DIRECTION('ref_axis',(0.,0.,-1.));
#16355=DIRECTION('',(0.,1.,0.));
#16356=DIRECTION('center_axis',(-1.,0.,0.));
#16357=DIRECTION('ref_axis',(0.,0.,-1.));
#16358=DIRECTION('center_axis',(0.,0.,-1.));
#16359=DIRECTION('ref_axis',(-1.,0.,0.));
#16360=DIRECTION('',(0.,1.,0.));
#16361=DIRECTION('',(1.,0.,0.));
#16362=DIRECTION('center_axis',(0.,0.707106781186548,-0.707106781186548));
#16363=DIRECTION('ref_axis',(-1.,0.,0.));
#16364=DIRECTION('',(-1.,0.,0.));
#16365=DIRECTION('',(0.,0.707106781186547,0.707106781186547));
#16366=DIRECTION('',(1.,0.,0.));
#16367=DIRECTION('',(-0.577350269189626,-0.577350269189626,-0.577350269189626));
#16368=DIRECTION('center_axis',(-0.707106781186548,-0.707106781186548,0.));
#16369=DIRECTION('ref_axis',(0.,0.,1.));
#16370=DIRECTION('',(0.,0.,-1.));
#16371=DIRECTION('',(0.707106781186547,-0.707106781186547,0.));
#16372=DIRECTION('',(0.,0.,1.));
#16373=DIRECTION('',(-0.577350269189625,0.577350269189625,-0.577350269189627));
#16374=DIRECTION('center_axis',(0.,-0.707106781186548,-0.707106781186548));
#16375=DIRECTION('ref_axis',(-1.,0.,0.));
#16376=DIRECTION('',(-1.,0.,0.));
#16377=DIRECTION('',(0.,0.707106781186547,-0.707106781186547));
#16378=DIRECTION('',(1.,0.,0.));
#16379=DIRECTION('center_axis',(0.,1.,0.));
#16380=DIRECTION('ref_axis',(-0.707106781186549,0.,-0.707106781186546));
#16381=DIRECTION('',(-0.707106781186547,0.707106781186547,-8.17756488897799E-16));
#16382=DIRECTION('center_axis',(0.,-1.,0.));
#16383=DIRECTION('ref_axis',(-0.707106781186549,0.,-0.707106781186546));
#16384=DIRECTION('center_axis',(0.,1.,0.));
#16385=DIRECTION('ref_axis',(-0.707106781186549,0.,-0.707106781186546));
#16386=DIRECTION('center_axis',(-0.707106781186548,-0.707106781186548,0.));
#16387=DIRECTION('ref_axis',(0.,0.,1.));
#16388=DIRECTION('',(-0.577350269189626,0.577350269189626,-0.577350269189626));
#16389=DIRECTION('',(0.,0.,-1.));
#16390=DIRECTION('',(0.,0.,1.));
#16391=DIRECTION('',(-0.577350269189626,0.577350269189626,0.577350269189625));
#16392=DIRECTION('center_axis',(1.,0.,0.));
#16393=DIRECTION('ref_axis',(0.,-0.707106781186547,-0.707106781186548));
#16394=DIRECTION('',(0.707106781186551,-4.08878244448901E-16,-0.707106781186544));
#16395=DIRECTION('center_axis',(-1.,0.,0.));
#16396=DIRECTION('ref_axis',(0.,-0.707106781186547,-0.707106781186548));
#16397=DIRECTION('center_axis',(1.,0.,0.));
#16398=DIRECTION('ref_axis',(0.,-0.707106781186547,-0.707106781186548));
#16399=DIRECTION('center_axis',(-0.707106781186548,0.,-0.707106781186548));
#16400=DIRECTION('ref_axis',(-0.707106781186548,0.,0.707106781186548));
#16401=DIRECTION('',(0.707106781186547,0.,-0.707106781186547));
#16402=DIRECTION('',(0.,-1.,0.));
#16403=DIRECTION('',(0.,1.,0.));
#16404=DIRECTION('center_axis',(1.,0.,0.));
#16405=DIRECTION('ref_axis',(0.,0.707106781186547,-0.707106781186548));
#16406=DIRECTION('',(0.707106781186549,0.707106781186546,0.));
#16407=DIRECTION('center_axis',(-1.,0.,0.));
#16408=DIRECTION('ref_axis',(0.,0.707106781186547,-0.707106781186548));
#16409=DIRECTION('center_axis',(1.,0.,0.));
#16410=DIRECTION('ref_axis',(0.,0.707106781186547,-0.707106781186548));
#16411=DIRECTION('center_axis',(-0.707106781186548,0.707106781186548,0.));
#16412=DIRECTION('ref_axis',(0.,0.,1.));
#16413=DIRECTION('',(0.,0.,-1.));
#16414=DIRECTION('',(0.,0.,1.));
#16415=DIRECTION('center_axis',(0.,-1.,0.));
#16416=DIRECTION('ref_axis',(-0.707106781186549,0.,-0.707106781186546));
#16417=DIRECTION('center_axis',(0.,1.,0.));
#16418=DIRECTION('ref_axis',(-0.707106781186549,0.,-0.707106781186546));
#16419=DIRECTION('',(0.707106781186547,0.707106781186547,8.17756488897799E-16));
#16420=DIRECTION('center_axis',(0.,-1.,0.));
#16421=DIRECTION('ref_axis',(-0.707106781186549,0.,-0.707106781186546));
#16422=DIRECTION('center_axis',(-0.707106781186548,0.707106781186548,0.));
#16423=DIRECTION('ref_axis',(0.,0.,1.));
#16424=DIRECTION('',(0.577350269189626,0.577350269189626,-0.577350269189625));
#16425=DIRECTION('',(0.,0.,-1.));
#16426=DIRECTION('',(0.,0.,1.));
#16427=DIRECTION('',(0.577350269189626,0.577350269189626,0.577350269189626));
#16428=DIRECTION('center_axis',(0.,1.,0.));
#16429=DIRECTION('ref_axis',(1.,0.,0.));
#16430=DIRECTION('',(-1.,0.,0.));
#16431=DIRECTION('center_axis',(0.,1.,0.));
#16432=DIRECTION('ref_axis',(1.,0.,0.));
#16433=DIRECTION('',(-1.,0.,0.));
#16434=DIRECTION('',(0.,0.,1.));
#16435=DIRECTION('',(-1.,0.,0.));
#16436=DIRECTION('',(0.,0.,-1.));
#16437=DIRECTION('',(-1.,0.,0.));
#16438=DIRECTION('center_axis',(0.,1.,0.));
#16439=DIRECTION('ref_axis',(0.707106781186546,0.,-0.707106781186549));
#16440=DIRECTION('',(0.,0.,-1.));
#16441=DIRECTION('',(1.,0.,0.));
#16442=DIRECTION('center_axis',(0.,-1.,0.));
#16443=DIRECTION('ref_axis',(1.,0.,0.));
#16444=DIRECTION('',(1.,0.,0.));
#16445=DIRECTION('',(-1.,0.,0.));
#16446=DIRECTION('center_axis',(-1.,0.,0.));
#16447=DIRECTION('ref_axis',(0.,-0.707106781186547,-0.707106781186548));
#16448=DIRECTION('',(1.,0.,0.));
#16449=DIRECTION('center_axis',(0.,0.,-1.));
#16450=DIRECTION('ref_axis',(-1.,0.,0.));
#16451=DIRECTION('',(-1.,0.,0.));
#16452=DIRECTION('center_axis',(-1.,0.,0.));
#16453=DIRECTION('ref_axis',(0.,0.707106781186547,-0.707106781186548));
#16454=DIRECTION('',(1.,0.,0.));
#16455=DIRECTION('center_axis',(0.,1.,0.));
#16456=DIRECTION('ref_axis',(1.,0.,0.));
#16457=DIRECTION('',(-1.,0.,0.));
#16458=DIRECTION('center_axis',(0.,1.,0.));
#16459=DIRECTION('ref_axis',(1.,0.,0.));
#16460=DIRECTION('',(-1.,0.,0.));
#16461=DIRECTION('',(0.,0.,1.));
#16462=DIRECTION('center_axis',(0.,-1.,0.));
#16463=DIRECTION('ref_axis',(0.707106781186546,0.,-0.707106781186549));
#16464=DIRECTION('',(1.,0.,0.));
#16465=DIRECTION('',(0.,0.,1.));
#16466=DIRECTION('',(1.,0.,0.));
#16467=DIRECTION('',(0.,0.,-1.));
#16468=DIRECTION('',(1.,0.,0.));
#16469=DIRECTION('center_axis',(0.,-1.,0.));
#16470=DIRECTION('ref_axis',(1.,0.,0.));
#16471=DIRECTION('center_axis',(0.,0.707106781186547,0.707106781186548));
#16472=DIRECTION('ref_axis',(1.,0.,0.));
#16473=DIRECTION('',(-0.577350269189626,0.577350269189626,-0.577350269189625));
#16474=DIRECTION('',(1.,0.,0.));
#16475=DIRECTION('',(0.591591578932266,0.570096221587387,-0.570096221587386));
#16476=DIRECTION('center_axis',(0.,0.707106781186548,-0.707106781186548));
#16477=DIRECTION('ref_axis',(-1.,0.,0.));
#16478=DIRECTION('',(0.577350269189626,0.577350269189626,0.577350269189626));
#16479=DIRECTION('',(-1.,0.,0.));
#16480=DIRECTION('center_axis',(0.,0.,-1.));
#16481=DIRECTION('ref_axis',(-1.,0.,0.));
#16482=DIRECTION('',(0.,1.,0.));
#16483=DIRECTION('',(1.,0.,0.));
#16484=DIRECTION('',(0.,1.,0.));
#16485=DIRECTION('center_axis',(0.577350269189626,0.577350269189626,0.577350269189626));
#16486=DIRECTION('ref_axis',(0.707106781186548,0.,-0.707106781186547));
#16487=DIRECTION('',(0.,0.707106781186548,-0.707106781186547));
#16488=DIRECTION('',(-0.707106781186548,0.,0.707106781186547));
#16489=DIRECTION('',(0.707106781186547,-0.707106781186547,0.));
#16490=DIRECTION('center_axis',(0.707106781186547,0.,0.707106781186548));
#16491=DIRECTION('ref_axis',(0.707106781186548,0.,-0.707106781186547));
#16492=DIRECTION('',(0.577350269189626,0.577350269189626,-0.577350269189625));
#16493=DIRECTION('',(0.,1.,0.));
#16494=DIRECTION('',(0.,-1.,0.));
#16495=DIRECTION('',(0.577350269189626,-0.577350269189626,-0.577350269189625));
#16496=DIRECTION('center_axis',(0.707106781186548,0.707106781186548,0.));
#16497=DIRECTION('ref_axis',(0.,0.,-1.));
#16498=DIRECTION('',(-0.707106781186547,0.707106781186547,0.));
#16499=DIRECTION('',(0.,0.,-1.));
#16500=DIRECTION('center_axis',(0.,-1.,0.));
#16501=DIRECTION('ref_axis',(0.707106781186546,0.,-0.707106781186549));
#16502=DIRECTION('center_axis',(0.,1.,0.));
#16503=DIRECTION('ref_axis',(0.707106781186546,0.,-0.707106781186549));
#16504=DIRECTION('',(0.,0.707106781186545,0.70710678118655));
#16505=DIRECTION('center_axis',(0.,0.707106781186548,-0.707106781186548));
#16506=DIRECTION('ref_axis',(-1.,0.,0.));
#16507=DIRECTION('',(0.577350269189626,-0.577350269189626,-0.577350269189626));
#16508=DIRECTION('',(-1.,0.,0.));
#16509=DIRECTION('center_axis',(0.,0.707106781186547,0.707106781186548));
#16510=DIRECTION('ref_axis',(1.,0.,0.));
#16511=DIRECTION('',(0.591591578932266,-0.570096221587387,0.570096221587386));
#16512=DIRECTION('',(1.,0.,0.));
#16513=DIRECTION('center_axis',(0.,1.,0.));
#16514=DIRECTION('ref_axis',(0.707106781186546,0.,-0.707106781186549));
#16515=DIRECTION('',(0.,-1.,0.));
#16516=DIRECTION('center_axis',(0.,-1.,0.));
#16517=DIRECTION('ref_axis',(0.707106781186546,0.,-0.707106781186549));
#16518=DIRECTION('',(0.,1.,0.));
#16519=DIRECTION('center_axis',(1.,0.,0.));
#16520=DIRECTION('ref_axis',(0.,0.,-1.));
#16521=DIRECTION('',(0.,0.,1.));
#16522=DIRECTION('center_axis',(0.707106781186548,-0.707106781186548,0.));
#16523=DIRECTION('ref_axis',(0.,0.,-1.));
#16524=DIRECTION('',(0.577350269189626,0.577350269189626,0.577350269189625));
#16525=DIRECTION('',(0.707106781186547,0.707106781186547,0.));
#16526=DIRECTION('center_axis',(0.,-0.707106781186547,0.707106781186548));
#16527=DIRECTION('ref_axis',(1.,0.,0.));
#16528=DIRECTION('',(-1.,0.,0.));
#16529=DIRECTION('',(-0.591591578932266,-0.570096221587387,-0.570096221587386));
#16530=DIRECTION('center_axis',(0.,0.,1.));
#16531=DIRECTION('ref_axis',(1.,0.,0.));
#16532=DIRECTION('',(0.,1.,0.));
#16533=DIRECTION('center_axis',(0.,0.,-1.));
#16534=DIRECTION('ref_axis',(1.,0.,0.));
#16535=DIRECTION('center_axis',(-0.693904010166723,0.,0.720067513969725));
#16536=DIRECTION('ref_axis',(0.720067513969725,0.,0.693904010166723));
#16537=DIRECTION('',(0.,-1.,0.));
#16538=DIRECTION('center_axis',(0.,1.,0.));
#16539=DIRECTION('ref_axis',(0.707106781186546,0.,-0.707106781186549));
#16540=DIRECTION('',(0.,0.707106781186545,-0.70710678118655));
#16541=DIRECTION('center_axis',(0.,-0.707106781186548,-0.707106781186548));
#16542=DIRECTION('ref_axis',(-1.,0.,0.));
#16543=DIRECTION('',(1.,0.,0.));
#16544=DIRECTION('',(0.577350269189625,0.577350269189625,-0.577350269189627));
#16545=DIRECTION('center_axis',(0.707106781186548,0.707106781186548,0.));
#16546=DIRECTION('ref_axis',(0.,0.,-1.));
#16547=DIRECTION('',(0.,0.,-1.));
#16548=DIRECTION('',(-0.707106781186547,0.707106781186547,0.));
#16549=DIRECTION('center_axis',(-1.,0.,0.));
#16550=DIRECTION('ref_axis',(0.,0.707106781186547,-0.707106781186548));
#16551=DIRECTION('',(-0.707106781186551,4.08878244448901E-16,-0.707106781186544));
#16552=DIRECTION('center_axis',(1.,0.,0.));
#16553=DIRECTION('ref_axis',(0.,0.707106781186547,-0.707106781186548));
#16554=DIRECTION('center_axis',(-1.,0.,0.));
#16555=DIRECTION('ref_axis',(0.,0.707106781186547,-0.707106781186548));
#16556=DIRECTION('center_axis',(0.707106781186548,0.,-0.707106781186548));
#16557=DIRECTION('ref_axis',(-0.707106781186548,0.,-0.707106781186548));
#16558=DIRECTION('',(0.,-1.,0.));
#16559=DIRECTION('',(-0.707106781186547,0.,-0.707106781186547));
#16560=DIRECTION('',(0.,1.,0.));
#16561=DIRECTION('center_axis',(-1.,0.,0.));
#16562=DIRECTION('ref_axis',(0.,-0.707106781186547,-0.707106781186548));
#16563=DIRECTION('',(-0.707106781186549,-0.707106781186546,0.));
#16564=DIRECTION('center_axis',(1.,0.,0.));
#16565=DIRECTION('ref_axis',(0.,-0.707106781186547,-0.707106781186548));
#16566=DIRECTION('center_axis',(-1.,0.,0.));
#16567=DIRECTION('ref_axis',(0.,-0.707106781186547,-0.707106781186548));
#16568=DIRECTION('center_axis',(0.707106781186548,-0.707106781186548,0.));
#16569=DIRECTION('ref_axis',(0.,0.,-1.));
#16570=DIRECTION('',(0.,0.,1.));
#16571=DIRECTION('center_axis',(0.,0.,-1.));
#16572=DIRECTION('ref_axis',(-1.,0.,0.));
#16573=DIRECTION('',(0.,1.,0.));
#16574=DIRECTION('center_axis',(0.,0.,1.));
#16575=DIRECTION('ref_axis',(1.,0.,0.));
#16576=DIRECTION('center_axis',(1.,0.,0.));
#16577=DIRECTION('ref_axis',(0.,0.,-1.));
#16578=DIRECTION('center_axis',(-1.,0.,0.));
#16579=DIRECTION('ref_axis',(0.,0.,-1.));
#16580=DIRECTION('center_axis',(-0.707106781186548,-0.707106781186548,0.));
#16581=DIRECTION('ref_axis',(0.,0.,1.));
#16582=DIRECTION('',(0.,0.,-1.));
#16583=DIRECTION('',(0.707106781186547,-0.707106781186547,0.));
#16584=DIRECTION('',(-0.577350269189626,0.577350269189626,-0.577350269189626));
#16585=DIRECTION('center_axis',(0.,-0.707106781186548,-0.707106781186548));
#16586=DIRECTION('ref_axis',(-1.,0.,0.));
#16587=DIRECTION('center_axis',(1.,0.,0.));
#16588=DIRECTION('ref_axis',(0.,-0.707106781186547,-0.707106781186548));
#16589=DIRECTION('',(0.707106781186551,-4.08878244448901E-16,-0.707106781186544));
#16590=DIRECTION('center_axis',(-1.,0.,0.));
#16591=DIRECTION('ref_axis',(0.,-0.707106781186547,-0.707106781186548));
#16592=DIRECTION('center_axis',(1.,0.,0.));
#16593=DIRECTION('ref_axis',(0.,-0.707106781186547,-0.707106781186548));
#16594=DIRECTION('center_axis',(-0.707106781186548,0.,-0.707106781186548));
#16595=DIRECTION('ref_axis',(-0.707106781186548,0.,0.707106781186548));
#16596=DIRECTION('',(0.707106781186547,0.,-0.707106781186547));
#16597=DIRECTION('',(0.,-1.,0.));
#16598=DIRECTION('',(0.,1.,0.));
#16599=DIRECTION('center_axis',(1.,0.,0.));
#16600=DIRECTION('ref_axis',(0.,0.707106781186547,-0.707106781186548));
#16601=DIRECTION('',(0.707106781186549,0.707106781186546,0.));
#16602=DIRECTION('center_axis',(-1.,0.,0.));
#16603=DIRECTION('ref_axis',(0.,0.707106781186547,-0.707106781186548));
#16604=DIRECTION('center_axis',(1.,0.,0.));
#16605=DIRECTION('ref_axis',(0.,0.707106781186547,-0.707106781186548));
#16606=DIRECTION('center_axis',(-0.707106781186548,0.707106781186548,0.));
#16607=DIRECTION('ref_axis',(0.,0.,1.));
#16608=DIRECTION('',(0.,0.,1.));
#16609=DIRECTION('center_axis',(-1.,0.,0.));
#16610=DIRECTION('ref_axis',(0.,0.,1.));
#16611=DIRECTION('center_axis',(1.,0.,0.));
#16612=DIRECTION('ref_axis',(0.,0.,-1.));
#16613=DIRECTION('center_axis',(0.,-0.707106781186548,-0.707106781186548));
#16614=DIRECTION('ref_axis',(-1.,0.,0.));
#16615=DIRECTION('center_axis',(0.,-0.707106781186547,0.707106781186548));
#16616=DIRECTION('ref_axis',(1.,0.,0.));
#16617=DIRECTION('',(-0.591591578932266,0.570096221587387,0.570096221587386));
#16618=DIRECTION('',(-1.,0.,0.));
#16619=DIRECTION('',(-0.577350269189626,-0.577350269189626,-0.577350269189625));
#16620=DIRECTION('center_axis',(-0.707106781186547,0.,0.707106781186548));
#16621=DIRECTION('ref_axis',(0.707106781186548,0.,0.707106781186547));
#16622=DIRECTION('',(0.,1.,0.));
#16623=DIRECTION('',(0.,-1.,0.));
#16624=DIRECTION('center_axis',(0.,-1.,0.));
#16625=DIRECTION('ref_axis',(1.,0.,0.));
#16626=DIRECTION('center_axis',(0.,1.,0.));
#16627=DIRECTION('ref_axis',(1.,0.,0.));
#16628=DIRECTION('center_axis',(-1.,0.,0.));
#16629=DIRECTION('ref_axis',(0.,0.,1.));
#16630=DIRECTION('',(0.,1.,0.));
#16631=DIRECTION('center_axis',(0.,1.,0.));
#16632=DIRECTION('ref_axis',(1.,0.,0.));
#16633=DIRECTION('center_axis',(0.,-1.,0.));
#16634=DIRECTION('ref_axis',(1.,0.,0.));
#16635=DIRECTION('center_axis',(0.,1.,0.));
#16636=DIRECTION('ref_axis',(1.,0.,0.));
#16637=DIRECTION('',(0.,1.,0.));
#16638=DIRECTION('',(0.,1.,0.));
#16639=DIRECTION('center_axis',(0.,-1.,0.));
#16640=DIRECTION('ref_axis',(1.,0.,0.));
#16641=DIRECTION('',(0.,-1.,0.));
#16642=DIRECTION('center_axis',(0.,1.,0.));
#16643=DIRECTION('ref_axis',(1.,0.,0.));
#16644=DIRECTION('center_axis',(0.693904010166723,0.,0.720067513969725));
#16645=DIRECTION('ref_axis',(0.720067513969725,0.,-0.693904010166723));
#16646=DIRECTION('',(0.,-1.,0.));
#16647=DIRECTION('center_axis',(0.993041625297607,0.,-0.117763875727185));
#16648=DIRECTION('ref_axis',(-0.117763875727185,0.,-0.993041625297607));
#16649=DIRECTION('',(0.,1.,0.));
#16650=DIRECTION('center_axis',(-0.993041625297607,0.,-0.117763875727185));
#16651=DIRECTION('ref_axis',(-0.117763875727185,0.,0.993041625297607));
#16652=DIRECTION('',(0.,-1.,0.));
#16653=DIRECTION('center_axis',(0.,-1.,0.));
#16654=DIRECTION('ref_axis',(1.,0.,0.));
#16655=DIRECTION('center_axis',(0.,-1.,0.));
#16656=DIRECTION('ref_axis',(1.,0.,0.));
#16657=DIRECTION('center_axis',(0.,1.,0.));
#16658=DIRECTION('ref_axis',(1.,0.,0.));
#16659=DIRECTION('center_axis',(0.,1.,0.));
#16660=DIRECTION('ref_axis',(1.,0.,0.));
#16661=DIRECTION('center_axis',(0.,1.,0.));
#16662=DIRECTION('ref_axis',(1.,0.,0.));
#16663=DIRECTION('',(-1.,0.,0.));
#16664=DIRECTION('',(0.,0.,1.));
#16665=DIRECTION('center_axis',(0.,-1.,0.));
#16666=DIRECTION('ref_axis',(1.,0.,0.));
#16667=DIRECTION('',(0.,0.,-1.));
#16668=DIRECTION('',(-1.,0.,0.));
#16669=DIRECTION('center_axis',(0.,0.,1.));
#16670=DIRECTION('ref_axis',(1.,0.,0.));
#16671=DIRECTION('',(1.,0.,0.));
#16672=DIRECTION('',(0.,1.,0.));
#16673=DIRECTION('center_axis',(0.55942034633874,0.,-0.828884115001756));
#16674=DIRECTION('ref_axis',(-0.828884115001756,0.,-0.55942034633874));
#16675=DIRECTION('',(0.,1.,0.));
#16676=DIRECTION('',(0.,-1.,0.));
#16677=DIRECTION('center_axis',(-0.55942034633874,0.,-0.828884115001756));
#16678=DIRECTION('ref_axis',(-0.828884115001756,0.,0.55942034633874));
#16679=DIRECTION('',(0.,-1.,0.));
#16680=DIRECTION('',(0.,1.,0.));
#16681=DIRECTION('center_axis',(0.,-1.,0.));
#16682=DIRECTION('ref_axis',(1.,0.,0.));
#16683=DIRECTION('center_axis',(0.,1.,0.));
#16684=DIRECTION('ref_axis',(1.,0.,0.));
#16685=DIRECTION('center_axis',(0.,1.,0.));
#16686=DIRECTION('ref_axis',(1.,0.,0.));
#16687=DIRECTION('center_axis',(0.,-1.,0.));
#16688=DIRECTION('ref_axis',(1.,0.,0.));
#16689=DIRECTION('center_axis',(0.,1.,0.));
#16690=DIRECTION('ref_axis',(1.,0.,0.));
#16691=DIRECTION('center_axis',(0.,1.,0.));
#16692=DIRECTION('ref_axis',(0.,0.,1.));
#16693=DIRECTION('',(1.,0.,0.));
#16694=DIRECTION('',(0.,0.,1.));
#16695=DIRECTION('',(0.,0.,-1.));
#16696=DIRECTION('center_axis',(1.,0.,0.));
#16697=DIRECTION('ref_axis',(0.,0.,-1.));
#16698=DIRECTION('center_axis',(0.,1.,0.));
#16699=DIRECTION('ref_axis',(1.,0.,0.));
#16700=DIRECTION('center_axis',(0.,1.,0.));
#16701=DIRECTION('ref_axis',(1.,0.,0.));
#16702=DIRECTION('center_axis',(0.,-1.,0.));
#16703=DIRECTION('ref_axis',(1.,0.,0.));
#16704=DIRECTION('center_axis',(0.,-1.,0.));
#16705=DIRECTION('ref_axis',(1.,0.,0.));
#16706=DIRECTION('center_axis',(0.,0.,1.));
#16707=DIRECTION('ref_axis',(1.,0.,0.));
#16708=DIRECTION('center_axis',(0.,0.,-1.));
#16709=DIRECTION('ref_axis',(1.,0.,0.));
#16710=DIRECTION('center_axis',(0.,1.,0.));
#16711=DIRECTION('ref_axis',(1.,0.,0.));
#16712=DIRECTION('center_axis',(-1.,0.,0.));
#16713=DIRECTION('ref_axis',(0.,0.,1.));
#16714=DIRECTION('',(0.,1.,0.));
#16715=DIRECTION('center_axis',(0.,0.,1.));
#16716=DIRECTION('ref_axis',(1.,0.,0.));
#16717=DIRECTION('center_axis',(0.,0.,-1.));
#16718=DIRECTION('ref_axis',(1.,0.,0.));
#16719=DIRECTION('',(0.,0.,-1.));
#16720=DIRECTION('center_axis',(0.,0.,-1.));
#16721=DIRECTION('ref_axis',(1.,0.,0.));
#16722=DIRECTION('',(0.,0.,-1.));
#16723=DIRECTION('center_axis',(0.,0.,1.));
#16724=DIRECTION('ref_axis',(1.,0.,0.));
#16725=DIRECTION('center_axis',(1.,0.,0.));
#16726=DIRECTION('ref_axis',(0.,0.,-1.));
#16727=DIRECTION('center_axis',(1.,0.,0.));
#16728=DIRECTION('ref_axis',(0.,0.,-1.));
#16729=DIRECTION('',(1.,0.,0.));
#16730=DIRECTION('center_axis',(-1.,0.,0.));
#16731=DIRECTION('ref_axis',(0.,0.,-1.));
#16732=DIRECTION('',(-1.,0.,0.));
#16733=DIRECTION('center_axis',(1.,0.,0.));
#16734=DIRECTION('ref_axis',(0.,-0.707106781186547,-0.707106781186548));
#16735=DIRECTION('',(1.,0.,0.));
#16736=DIRECTION('center_axis',(-1.,0.,0.));
#16737=DIRECTION('ref_axis',(0.,0.707106781186547,-0.707106781186548));
#16738=DIRECTION('',(-1.,0.,0.));
#16739=DIRECTION('center_axis',(0.,1.,0.));
#16740=DIRECTION('ref_axis',(-0.707106781186549,0.,-0.707106781186546));
#16741=DIRECTION('',(0.,-1.,0.));
#16742=DIRECTION('center_axis',(0.,0.,-1.));
#16743=DIRECTION('ref_axis',(-1.,0.,0.));
#16744=DIRECTION('',(0.,1.,0.));
#16745=DIRECTION('center_axis',(0.,0.,-1.));
#16746=DIRECTION('ref_axis',(-1.,0.,0.));
#16747=DIRECTION('center_axis',(-1.,0.,0.));
#16748=DIRECTION('ref_axis',(0.,0.,1.));
#19984=CARTESIAN_POINT('',(0.,0.,0.));
#19985=CARTESIAN_POINT('Origin',(-30.64,-5.76,-12.225));
#19986=CARTESIAN_POINT('',(-30.4,-5.52,-20.2));
#19987=CARTESIAN_POINT('',(-30.88,-6.,-19.72));
#19988=CARTESIAN_POINT('',(-28.6708476104047,-3.79084761040473,-21.9291523895953));
#19989=CARTESIAN_POINT('',(-30.88,-6.,-34.5));
#19990=CARTESIAN_POINT('',(-30.88,-6.,-12.225));
#19991=CARTESIAN_POINT('',(-30.4,-5.52,-34.5));
#19992=CARTESIAN_POINT('',(-30.88,-6.,-34.5));
#19993=CARTESIAN_POINT('',(-30.4,-5.52,-12.225));
#19994=CARTESIAN_POINT('Origin',(-30.64,-2.,-34.5));
#19995=CARTESIAN_POINT('',(-30.88,-2.,-38.5));
#19996=CARTESIAN_POINT('Origin',(-30.88,-2.,-34.5));
#19997=CARTESIAN_POINT('',(-30.4,-2.,-38.02));
#19998=CARTESIAN_POINT('',(-30.88,-2.,-38.5));
#19999=CARTESIAN_POINT('Origin',(-30.4,-2.,-34.5));
#20000=CARTESIAN_POINT('Origin',(-30.64,-6.,-38.26));
#20001=CARTESIAN_POINT('',(-30.88,2.,-38.5));
#20002=CARTESIAN_POINT('',(-30.4,2.,-38.02));
#20003=CARTESIAN_POINT('',(-30.88,2.,-38.5));
#20004=CARTESIAN_POINT('',(-30.4,-6.,-38.02));
#20005=CARTESIAN_POINT('',(-30.88,-6.,-38.5));
#20006=CARTESIAN_POINT('Origin',(-30.64,2.,-34.5));
#20007=CARTESIAN_POINT('',(-30.88,6.,-34.5));
#20008=CARTESIAN_POINT('Origin',(-30.88,2.,-34.5));
#20009=CARTESIAN_POINT('',(-30.4,5.52,-34.5));
#20010=CARTESIAN_POINT('',(-30.88,6.,-34.5));
#20011=CARTESIAN_POINT('Origin',(-30.4,2.,-34.5));
#20012=CARTESIAN_POINT('Origin',(-30.64,5.76,-12.225));
#20013=CARTESIAN_POINT('',(-30.4,5.52,-20.2));
#20014=CARTESIAN_POINT('',(-30.4,5.52,-12.225));
#20015=CARTESIAN_POINT('',(-30.88,6.,-19.72));
#20016=CARTESIAN_POINT('',(-30.88,6.,-12.225));
#20017=CARTESIAN_POINT('',(-30.88,6.,-19.72));
#20018=CARTESIAN_POINT('Origin',(-11.0900856624284,5.76,-19.96));
#20019=CARTESIAN_POINT('',(-21.9401823146482,6.,-19.72));
#20020=CARTESIAN_POINT('',(-11.0900856624284,6.,-19.72));
#20021=CARTESIAN_POINT('',(-22.1531126481134,5.52,-20.2));
#20022=CARTESIAN_POINT('Ctrl Pts',(-22.1531126481134,5.52,-20.2));
#20023=CARTESIAN_POINT('Ctrl Pts',(-22.0466474813905,5.76115898072722,-19.9588410192728));
#20024=CARTESIAN_POINT('Ctrl Pts',(-21.9401823146482,6.,-19.72));
#20025=CARTESIAN_POINT('',(-11.0900856624284,5.52,-20.2));
#20026=CARTESIAN_POINT('Origin',(-30.4,-6.,-20.2));
#20027=CARTESIAN_POINT('',(-30.4,-6.,-20.2));
#20028=CARTESIAN_POINT('',(-30.4,2.63299061816681E-16,-30.85));
#20029=CARTESIAN_POINT('Origin',(-30.4,0.,-33.));
#20030=CARTESIAN_POINT('Origin',(-22.1801713248568,-6.,-20.2));
#20031=CARTESIAN_POINT('',(-22.1801713248568,5.5,-20.2));
#20032=CARTESIAN_POINT('Ctrl Pts',(-22.1531126481135,5.51999999999993,-20.2));
#20033=CARTESIAN_POINT('Ctrl Pts',(-22.1666374752019,5.51000610346768,-20.2));
#20034=CARTESIAN_POINT('Ctrl Pts',(-22.1801713248568,5.5,-20.2));
#20035=CARTESIAN_POINT('',(-22.1801713248568,-5.5,-20.2));
#20036=CARTESIAN_POINT('',(-22.1801713248568,-6.,-20.2));
#20037=CARTESIAN_POINT('',(-22.1531126481134,-5.52,-20.2));
#20038=CARTESIAN_POINT('Ctrl Pts',(-22.1801713248568,-5.5,-20.2));
#20039=CARTESIAN_POINT('Ctrl Pts',(-22.1666374752019,-5.51000610346768,
-20.2));
#20040=CARTESIAN_POINT('Ctrl Pts',(-22.1531126481134,-5.51999999999993,
-20.2));
#20041=CARTESIAN_POINT('',(-11.0900856624284,-5.52,-20.2));
#20042=CARTESIAN_POINT('Origin',(-17.2,5.76,-5.76));
#20043=CARTESIAN_POINT('',(-34.4,5.52,-6.));
#20044=CARTESIAN_POINT('',(-43.65,5.52,-6.));
#20045=CARTESIAN_POINT('',(-17.2,5.52,-6.));
#20046=CARTESIAN_POINT('',(-43.65,6.,-5.52));
#20047=CARTESIAN_POINT('',(-43.65,5.52,-6.));
#20048=CARTESIAN_POINT('',(-33.92,6.,-5.52));
#20049=CARTESIAN_POINT('',(-17.2,6.,-5.52));
#20050=CARTESIAN_POINT('',(-33.92,6.,-5.52));
#20051=CARTESIAN_POINT('Origin',(-34.16,-5.76,-21.375));
#20052=CARTESIAN_POINT('',(-34.4,-5.52,-6.));
#20053=CARTESIAN_POINT('',(-34.4,-5.52,-34.5));
#20054=CARTESIAN_POINT('',(-34.4,-5.52,-21.375));
#20055=CARTESIAN_POINT('',(-33.92,-6.,-34.5));
#20056=CARTESIAN_POINT('',(-34.4,-5.52,-34.5));
#20057=CARTESIAN_POINT('',(-33.92,-6.,-5.52));
#20058=CARTESIAN_POINT('',(-33.92,-6.,-21.375));
#20059=CARTESIAN_POINT('',(-33.92,-6.,-5.52));
#20060=CARTESIAN_POINT('Origin',(-17.2,-5.76,-5.76));
#20061=CARTESIAN_POINT('',(-43.65,-6.,-5.52));
#20062=CARTESIAN_POINT('',(-17.2,-6.,-5.52));
#20063=CARTESIAN_POINT('',(-43.65,-5.52,-6.));
#20064=CARTESIAN_POINT('',(-43.65,-6.,-5.52));
#20065=CARTESIAN_POINT('',(-17.2,-5.52,-6.));
#20066=CARTESIAN_POINT('Origin',(-43.65,-5.76,-4.));
#20067=CARTESIAN_POINT('',(-45.17,-6.,-4.));
#20068=CARTESIAN_POINT('',(-45.65,-5.52,-4.));
#20069=CARTESIAN_POINT('',(-45.17,-6.,-4.));
#20070=CARTESIAN_POINT('Origin',(-43.65,-5.52,-4.));
#20071=CARTESIAN_POINT('Origin',(-43.65,-6.,-4.));
#20072=CARTESIAN_POINT('Origin',(-45.41,-5.76,-5.125));
#20073=CARTESIAN_POINT('',(-45.41,-5.76,-0.74));
#20074=CARTESIAN_POINT('',(-45.65,-5.52,-0.98));
#20075=CARTESIAN_POINT('',(-46.1008333333333,-5.06916666666667,-1.43083333333333));
#20076=CARTESIAN_POINT('',(-45.65,-5.52,-5.125));
#20077=CARTESIAN_POINT('',(-45.17,-6.,-0.98));
#20078=CARTESIAN_POINT('',(-45.17,-6.,-5.125));
#20079=CARTESIAN_POINT('',(-34.6111805796715,-16.5588194203284,-11.5388194203284));
#20080=CARTESIAN_POINT('Origin',(-34.16,-2.,-34.5));
#20081=CARTESIAN_POINT('',(-34.4,-2.,-38.02));
#20082=CARTESIAN_POINT('',(-33.92,-2.,-38.5));
#20083=CARTESIAN_POINT('',(-34.4,-2.,-38.02));
#20084=CARTESIAN_POINT('Origin',(-33.92,-2.,-34.5));
#20085=CARTESIAN_POINT('Origin',(-34.4,-2.,-34.5));
#20086=CARTESIAN_POINT('Origin',(-34.16,-6.,-38.26));
#20087=CARTESIAN_POINT('',(-34.4,2.,-38.02));
#20088=CARTESIAN_POINT('',(-33.92,2.,-38.5));
#20089=CARTESIAN_POINT('',(-34.4,2.,-38.02));
#20090=CARTESIAN_POINT('',(-33.92,-6.,-38.5));
#20091=CARTESIAN_POINT('',(-34.4,-6.,-38.02));
#20092=CARTESIAN_POINT('Origin',(-34.16,2.,-34.5));
#20093=CARTESIAN_POINT('',(-34.4,5.52,-34.5));
#20094=CARTESIAN_POINT('',(-33.92,6.,-34.5));
#20095=CARTESIAN_POINT('',(-34.4,5.52,-34.5));
#20096=CARTESIAN_POINT('Origin',(-33.92,2.,-34.5));
#20097=CARTESIAN_POINT('Origin',(-34.4,2.,-34.5));
#20098=CARTESIAN_POINT('Origin',(-34.16,5.76,-21.375));
#20099=CARTESIAN_POINT('',(-33.92,6.,-21.375));
#20100=CARTESIAN_POINT('',(-34.4,5.52,-21.375));
#20101=CARTESIAN_POINT('Origin',(-43.65,5.76,-4.));
#20102=CARTESIAN_POINT('',(-45.65,5.52,-4.));
#20103=CARTESIAN_POINT('Origin',(-43.65,5.52,-4.));
#20104=CARTESIAN_POINT('',(-45.17,6.,-4.));
#20105=CARTESIAN_POINT('',(-45.65,5.52,-4.));
#20106=CARTESIAN_POINT('Origin',(-43.65,6.,-4.));
#20107=CARTESIAN_POINT('Origin',(-45.41,5.76,-5.125));
#20108=CARTESIAN_POINT('',(-45.41,5.76,-0.74));
#20109=CARTESIAN_POINT('',(-45.17,6.,-0.98));
#20110=CARTESIAN_POINT('',(-34.6111805796715,16.5588194203284,-11.5388194203284));
#20111=CARTESIAN_POINT('',(-45.17,6.,-5.125));
#20112=CARTESIAN_POINT('',(-45.65,5.52,-0.98));
#20113=CARTESIAN_POINT('',(-45.65,5.52,-5.125));
#20114=CARTESIAN_POINT('',(-48.1008333333333,3.06916666666667,-3.43083333333333));
#20115=CARTESIAN_POINT('Origin',(0.,-6.,-4.25));
#20116=CARTESIAN_POINT('',(-21.9401823146482,-6.,-19.72));
#20117=CARTESIAN_POINT('',(-11.0900856624284,-6.,-19.72));
#20118=CARTESIAN_POINT('',(21.9401823146482,-6.,-19.72));
#20119=CARTESIAN_POINT('Origin',(0.,-6.,0.));
#20120=CARTESIAN_POINT('',(30.88,-6.,-19.72));
#20121=CARTESIAN_POINT('',(15.2,-6.,-19.72));
#20122=CARTESIAN_POINT('',(30.88,-6.,-34.5));
#20123=CARTESIAN_POINT('',(30.88,-6.,-21.375));
#20124=CARTESIAN_POINT('',(33.92,-6.,-34.5));
#20125=CARTESIAN_POINT('',(17.2,-6.,-34.5));
#20126=CARTESIAN_POINT('',(33.92,-6.,-5.52));
#20127=CARTESIAN_POINT('',(33.92,-6.,-5.125));
#20128=CARTESIAN_POINT('',(43.65,-6.,-5.52));
#20129=CARTESIAN_POINT('',(22.825,-6.,-5.52));
#20130=CARTESIAN_POINT('',(45.17,-6.,-4.));
#20131=CARTESIAN_POINT('Origin',(43.65,-6.,-4.));
#20132=CARTESIAN_POINT('',(45.17,-6.,-0.98));
#20133=CARTESIAN_POINT('',(45.17,-6.,-2.375));
#20134=CARTESIAN_POINT('',(20.4765622114651,-6.,-0.98));
#20135=CARTESIAN_POINT('',(14.9979165219706,-6.,-0.98));
#20136=CARTESIAN_POINT('',(-20.4765622114651,-6.,-0.98));
#20137=CARTESIAN_POINT('Origin',(0.,-6.,0.));
#20138=CARTESIAN_POINT('',(14.9979165219706,-6.,-0.98));
#20139=CARTESIAN_POINT('',(-15.2,-6.,-34.5));
#20140=CARTESIAN_POINT('Origin',(-15.2,-2.,-34.5));
#20141=CARTESIAN_POINT('',(-15.2,-2.,-38.5));
#20142=CARTESIAN_POINT('Origin',(-30.4,-6.,-38.5));
#20143=CARTESIAN_POINT('',(-15.2,2.,-38.5));
#20144=CARTESIAN_POINT('Origin',(-15.2,2.,-34.5));
#20145=CARTESIAN_POINT('',(-15.2,6.,-34.5));
#20146=CARTESIAN_POINT('Origin',(0.,6.,-4.25));
#20147=CARTESIAN_POINT('',(-20.4765622114651,6.,-0.98));
#20148=CARTESIAN_POINT('',(14.9979165219706,6.,-0.98));
#20149=CARTESIAN_POINT('',(20.4765622114651,6.,-0.98));
#20150=CARTESIAN_POINT('Origin',(0.,6.,0.));
#20151=CARTESIAN_POINT('',(45.17,6.,-0.98));
#20152=CARTESIAN_POINT('',(14.9979165219706,6.,-0.98));
#20153=CARTESIAN_POINT('',(45.17,6.,-4.));
#20154=CARTESIAN_POINT('',(45.17,6.,-2.375));
#20155=CARTESIAN_POINT('',(43.65,6.,-5.52));
#20156=CARTESIAN_POINT('Origin',(43.65,6.,-4.));
#20157=CARTESIAN_POINT('',(33.92,6.,-5.52));
#20158=CARTESIAN_POINT('',(22.825,6.,-5.52));
#20159=CARTESIAN_POINT('',(33.92,6.,-34.5));
#20160=CARTESIAN_POINT('',(33.92,6.,-5.125));
#20161=CARTESIAN_POINT('',(30.88,6.,-34.5));
#20162=CARTESIAN_POINT('',(17.2,6.,-34.5));
#20163=CARTESIAN_POINT('',(30.88,6.,-19.72));
#20164=CARTESIAN_POINT('',(30.88,6.,-21.375));
#20165=CARTESIAN_POINT('',(21.9401823146482,6.,-19.72));
#20166=CARTESIAN_POINT('',(15.2,6.,-19.72));
#20167=CARTESIAN_POINT('Origin',(0.,6.,0.));
#20168=CARTESIAN_POINT('Origin',(14.9979165219706,5.76,-0.74));
#20169=CARTESIAN_POINT('',(-45.17,5.52,-0.5));
#20170=CARTESIAN_POINT('',(-45.17,5.52,-0.5));
#20171=CARTESIAN_POINT('',(-20.4737490231322,5.52,-0.5));
#20172=CARTESIAN_POINT('',(14.9979165219706,5.52,-0.5));
#20173=CARTESIAN_POINT('',(-20.2359894539709,5.74912062451896,-0.729120624518964));
#20174=CARTESIAN_POINT('',(-16.044254314835,9.78854993659521,-4.7685499365952));
#20175=CARTESIAN_POINT('Ctrl Pts',(-20.2359894539709,5.74912062451896,-0.729120624518964));
#20176=CARTESIAN_POINT('Ctrl Pts',(-20.3562758327179,5.87381908208973,-0.853819082089726));
#20177=CARTESIAN_POINT('Ctrl Pts',(-20.4765622114651,6.,-0.98));
#20178=CARTESIAN_POINT('Origin',(15.2,5.76,-19.96));
#20179=CARTESIAN_POINT('',(30.4,5.52,-20.2));
#20180=CARTESIAN_POINT('',(27.8308333333333,2.95083333333333,-22.7691666666667));
#20181=CARTESIAN_POINT('',(22.1531126481133,5.52,-20.2));
#20182=CARTESIAN_POINT('',(15.2,5.52,-20.2));
#20183=CARTESIAN_POINT('Ctrl Pts',(21.9401823146482,6.,-19.72));
#20184=CARTESIAN_POINT('Ctrl Pts',(22.0466474813905,5.76115898072722,-19.9588410192728));
#20185=CARTESIAN_POINT('Ctrl Pts',(22.1531126481134,5.52,-20.2));
#20186=CARTESIAN_POINT('Origin',(30.4,-6.,-20.2));
#20187=CARTESIAN_POINT('',(30.4,-5.52,-20.2));
#20188=CARTESIAN_POINT('',(30.4,-6.,-20.2));
#20189=CARTESIAN_POINT('',(22.1531126481134,-5.52,-20.2));
#20190=CARTESIAN_POINT('',(15.2,-5.52,-20.2));
#20191=CARTESIAN_POINT('',(22.1801713248568,-5.5,-20.2));
#20192=CARTESIAN_POINT('Ctrl Pts',(22.1531126481135,-5.51999999999993,-20.2));
#20193=CARTESIAN_POINT('Ctrl Pts',(22.1666374752019,-5.51000610346768,-20.2));
#20194=CARTESIAN_POINT('Ctrl Pts',(22.1801713248568,-5.5,-20.2));
#20195=CARTESIAN_POINT('',(22.1801713248568,5.5,-20.2));
#20196=CARTESIAN_POINT('',(22.1801713248568,-6.,-20.2));
#20197=CARTESIAN_POINT('Ctrl Pts',(22.1801713248568,5.5,-20.2));
#20198=CARTESIAN_POINT('Ctrl Pts',(22.1666374752019,5.51000610346769,-20.2));
#20199=CARTESIAN_POINT('Ctrl Pts',(22.1531126481135,5.51999999999993,-20.2));
#20200=CARTESIAN_POINT('Origin',(45.65,5.52,-0.98));
#20201=CARTESIAN_POINT('',(45.17,5.52,-0.5));
#20202=CARTESIAN_POINT('',(45.17,5.52,-0.5));
#20203=CARTESIAN_POINT('',(45.65,5.52,-0.98));
#20204=CARTESIAN_POINT('',(45.65,5.52,-0.98));
#20205=CARTESIAN_POINT('',(45.17,6.,-0.98));
#20206=CARTESIAN_POINT('Origin',(45.41,-6.,-0.74));
#20207=CARTESIAN_POINT('',(45.41,-5.76,-0.74));
#20208=CARTESIAN_POINT('',(45.65,-5.52,-0.98));
#20209=CARTESIAN_POINT('',(45.6425,-5.5275,-0.9725));
#20210=CARTESIAN_POINT('',(45.65,-6.,-0.98));
#20211=CARTESIAN_POINT('',(45.17,-5.52,-0.5));
#20212=CARTESIAN_POINT('',(45.17,-6.,-0.5));
#20213=CARTESIAN_POINT('',(40.3813194203284,-0.731319420328439,4.28868057967155));
#20214=CARTESIAN_POINT('Origin',(45.41,5.76,-2.375));
#20215=CARTESIAN_POINT('',(45.65,5.52,-4.));
#20216=CARTESIAN_POINT('',(45.65,5.52,-4.));
#20217=CARTESIAN_POINT('',(45.65,5.52,-2.375));
#20218=CARTESIAN_POINT('Origin',(43.65,5.76,-4.));
#20219=CARTESIAN_POINT('',(43.65,5.52,-6.));
#20220=CARTESIAN_POINT('Origin',(43.65,5.52,-4.));
#20221=CARTESIAN_POINT('',(43.65,5.52,-6.));
#20222=CARTESIAN_POINT('Origin',(22.825,5.76,-5.76));
#20223=CARTESIAN_POINT('',(34.4,5.52,-6.));
#20224=CARTESIAN_POINT('',(32.165,7.755,-3.765));
#20225=CARTESIAN_POINT('',(22.825,5.52,-6.));
#20226=CARTESIAN_POINT('Origin',(14.9979165219706,5.76,-0.74));
#20227=CARTESIAN_POINT('',(20.2359894539709,5.74912062451897,-0.729120624518967));
#20228=CARTESIAN_POINT('',(20.4737490231322,5.52,-0.5));
#20229=CARTESIAN_POINT('',(21.2932340819055,4.73029076090437,0.289709239095628));
#20230=CARTESIAN_POINT('',(14.9979165219706,5.52,-0.5));
#20231=CARTESIAN_POINT('Ctrl Pts',(20.4765622114651,6.,-0.98));
#20232=CARTESIAN_POINT('Ctrl Pts',(20.3562758327179,5.87381908208973,-0.853819082089731));
#20233=CARTESIAN_POINT('Ctrl Pts',(20.2359894539709,5.74912062451897,-0.729120624518967));
#20234=CARTESIAN_POINT('Origin',(43.65,-6.,-4.));
#20235=CARTESIAN_POINT('',(45.65,-5.52,-4.));
#20236=CARTESIAN_POINT('',(45.65,-6.,-4.));
#20237=CARTESIAN_POINT('',(43.65,-5.52,-6.));
#20238=CARTESIAN_POINT('Origin',(43.65,-5.52,-4.));
#20239=CARTESIAN_POINT('',(43.65,-6.,-6.));
#20240=CARTESIAN_POINT('Origin',(45.65,-6.,-0.5));
#20241=CARTESIAN_POINT('',(45.65,-5.52,-2.375));
#20242=CARTESIAN_POINT('Origin',(45.41,-5.76,-2.375));
#20243=CARTESIAN_POINT('',(45.17,-6.,-0.98));
#20244=CARTESIAN_POINT('',(45.17,-6.,-4.));
#20245=CARTESIAN_POINT('Origin',(14.9979165219706,-5.76,-0.74));
#20246=CARTESIAN_POINT('',(20.4737490231322,-5.52,-0.5));
#20247=CARTESIAN_POINT('',(14.9979165219706,-5.52,-0.5));
#20248=CARTESIAN_POINT('',(20.2359894539709,-5.74912062451896,-0.729120624518964));
#20249=CARTESIAN_POINT('',(19.2696493386723,-6.68034897211366,-1.66034897211366));
#20250=CARTESIAN_POINT('Ctrl Pts',(20.2359894539709,-5.74912062451896,-0.729120624518964));
#20251=CARTESIAN_POINT('Ctrl Pts',(20.356275832718,-5.87381908208986,-0.853819082089863));
#20252=CARTESIAN_POINT('Ctrl Pts',(20.4765622114651,-6.,-0.98));
#20253=CARTESIAN_POINT('Origin',(29.9958330439413,-6.,-0.5));
#20254=CARTESIAN_POINT('',(20.4737490231322,-6.,-0.5));
#20255=CARTESIAN_POINT('',(37.25,-2.75545529808154E-16,-0.5));
#20256=CARTESIAN_POINT('Origin',(39.5,0.,-0.5));
#20257=CARTESIAN_POINT('Origin',(20.2248703552884,-6.,-0.7398357130565));
#20258=CARTESIAN_POINT('',(19.9759916874447,5.5,-0.979671426113));
#20259=CARTESIAN_POINT('Ctrl Pts',(20.2359894539709,5.74912062451897,-0.729120624518967));
#20260=CARTESIAN_POINT('Ctrl Pts',(20.1051859468428,5.6229407173369,-0.855171413339672));
#20261=CARTESIAN_POINT('Ctrl Pts',(19.9759916874446,5.5,-0.979671426113002));
#20262=CARTESIAN_POINT('',(19.9759916874447,-5.5,-0.979671426113));
#20263=CARTESIAN_POINT('',(19.9759916874447,-6.,-0.979671426113));
#20264=CARTESIAN_POINT('Ctrl Pts',(19.9759916874447,-5.5,-0.979671426112999));
#20265=CARTESIAN_POINT('Ctrl Pts',(20.1051859468428,-5.62294071733695,-0.855171413339621));
#20266=CARTESIAN_POINT('Ctrl Pts',(20.2359894539709,-5.74912062451896,-0.729120624518964));
#20267=CARTESIAN_POINT('Origin',(43.65,-5.76,-4.));
#20268=CARTESIAN_POINT('',(43.65,-6.,-5.52));
#20269=CARTESIAN_POINT('Origin',(22.825,-5.76,-5.76));
#20270=CARTESIAN_POINT('',(34.4,-5.52,-6.));
#20271=CARTESIAN_POINT('',(22.825,-5.52,-6.));
#20272=CARTESIAN_POINT('',(33.92,-6.,-5.52));
#20273=CARTESIAN_POINT('Origin',(34.16,5.76,-5.125));
#20274=CARTESIAN_POINT('',(34.4,5.52,-34.5));
#20275=CARTESIAN_POINT('',(34.4,5.52,-5.125));
#20276=CARTESIAN_POINT('',(34.4,5.52,-34.5));
#20277=CARTESIAN_POINT('Origin',(34.16,2.,-34.5));
#20278=CARTESIAN_POINT('',(34.4,2.,-38.02));
#20279=CARTESIAN_POINT('',(33.92,2.,-38.5));
#20280=CARTESIAN_POINT('',(34.4,2.,-38.02));
#20281=CARTESIAN_POINT('Origin',(33.92,2.,-34.5));
#20282=CARTESIAN_POINT('Origin',(34.4,2.,-34.5));
#20283=CARTESIAN_POINT('Origin',(34.16,-6.,-38.26));
#20284=CARTESIAN_POINT('',(34.4,-2.,-38.02));
#20285=CARTESIAN_POINT('',(34.4,-6.,-38.02));
#20286=CARTESIAN_POINT('',(33.92,-2.,-38.5));
#20287=CARTESIAN_POINT('',(34.4,-2.,-38.02));
#20288=CARTESIAN_POINT('',(33.92,-6.,-38.5));
#20289=CARTESIAN_POINT('Origin',(34.16,-2.,-34.5));
#20290=CARTESIAN_POINT('',(34.4,-5.52,-34.5));
#20291=CARTESIAN_POINT('',(34.4,-5.52,-34.5));
#20292=CARTESIAN_POINT('Origin',(33.92,-2.,-34.5));
#20293=CARTESIAN_POINT('Origin',(34.4,-2.,-34.5));
#20294=CARTESIAN_POINT('Origin',(34.16,-5.76,-5.125));
#20295=CARTESIAN_POINT('',(34.4,-5.52,-5.125));
#20296=CARTESIAN_POINT('Origin',(45.65,-6.,-6.));
#20297=CARTESIAN_POINT('',(34.4,-6.,-6.));
#20298=CARTESIAN_POINT('',(37.25,-2.75545529808154E-16,-6.));
#20299=CARTESIAN_POINT('Origin',(39.5,0.,-6.));
#20300=CARTESIAN_POINT('Origin',(34.4,-6.,-6.));
#20301=CARTESIAN_POINT('',(34.4,-2.63299061816681E-16,-30.85));
#20302=CARTESIAN_POINT('Origin',(34.4,0.,-33.));
#20303=CARTESIAN_POINT('Origin',(30.64,-5.76,-21.375));
#20304=CARTESIAN_POINT('',(30.4,-5.52,-34.5));
#20305=CARTESIAN_POINT('',(30.4,-5.52,-21.375));
#20306=CARTESIAN_POINT('',(30.4,-5.52,-34.5));
#20307=CARTESIAN_POINT('',(30.88,-6.,-19.72));
#20308=CARTESIAN_POINT('Origin',(15.2,-5.76,-19.96));
#20309=CARTESIAN_POINT('Ctrl Pts',(22.1531126481134,-5.52,-20.2));
#20310=CARTESIAN_POINT('Ctrl Pts',(22.0466474813867,-5.76115898073578,-19.9588410192642));
#20311=CARTESIAN_POINT('Ctrl Pts',(21.9401823146482,-6.,-19.72));
#20312=CARTESIAN_POINT('Origin',(30.64,-2.,-34.5));
#20313=CARTESIAN_POINT('',(30.4,-2.,-38.02));
#20314=CARTESIAN_POINT('',(30.88,-2.,-38.5));
#20315=CARTESIAN_POINT('',(30.4,-2.,-38.02));
#20316=CARTESIAN_POINT('Origin',(30.88,-2.,-34.5));
#20317=CARTESIAN_POINT('Origin',(30.4,-2.,-34.5));
#20318=CARTESIAN_POINT('Origin',(30.64,-6.,-38.26));
#20319=CARTESIAN_POINT('',(30.4,2.,-38.02));
#20320=CARTESIAN_POINT('',(30.88,2.,-38.5));
#20321=CARTESIAN_POINT('',(30.4,2.,-38.02));
#20322=CARTESIAN_POINT('',(30.88,-6.,-38.5));
#20323=CARTESIAN_POINT('',(30.4,-6.,-38.02));
#20324=CARTESIAN_POINT('Origin',(30.64,2.,-34.5));
#20325=CARTESIAN_POINT('',(30.4,5.52,-34.5));
#20326=CARTESIAN_POINT('',(30.4,5.52,-34.5));
#20327=CARTESIAN_POINT('Origin',(30.88,2.,-34.5));
#20328=CARTESIAN_POINT('Origin',(30.4,2.,-34.5));
#20329=CARTESIAN_POINT('Origin',(30.64,5.76,-21.375));
#20330=CARTESIAN_POINT('',(30.4,5.52,-21.375));
#20331=CARTESIAN_POINT('Origin',(30.4,-6.,-38.5));
#20332=CARTESIAN_POINT('',(30.4,-2.63299061816681E-16,-30.85));
#20333=CARTESIAN_POINT('Origin',(30.4,0.,-33.));
#20334=CARTESIAN_POINT('Origin',(-11.0900856624284,-5.76,-19.96));
#20335=CARTESIAN_POINT('Ctrl Pts',(-21.9401823146482,-6.,-19.72));
#20336=CARTESIAN_POINT('Ctrl Pts',(-22.0466474813867,-5.76115898073578,
-19.9588410192642));
#20337=CARTESIAN_POINT('Ctrl Pts',(-22.1531126481134,-5.52,-20.2));
#20338=CARTESIAN_POINT('Origin',(14.9979165219706,-5.76,-0.74));
#20339=CARTESIAN_POINT('',(-20.2359894539709,-5.74912062451896,-0.729120624518966));
#20340=CARTESIAN_POINT('Ctrl Pts',(-20.4765622114651,-6.,-0.98));
#20341=CARTESIAN_POINT('Ctrl Pts',(-20.356275832718,-5.87381908208986,-0.853819082089866));
#20342=CARTESIAN_POINT('Ctrl Pts',(-20.2359894539709,-5.74912062451896,
-0.729120624518966));
#20343=CARTESIAN_POINT('',(-20.4737490231322,-5.52,-0.5));
#20344=CARTESIAN_POINT('',(-14.0206695716018,-11.7386081478045,-6.71860814780449));
#20345=CARTESIAN_POINT('',(-45.17,-5.52,-0.5));
#20346=CARTESIAN_POINT('',(14.9979165219706,-5.52,-0.5));
#20347=CARTESIAN_POINT('',(-45.17,-5.52,-0.5));
#20348=CARTESIAN_POINT('Origin',(-45.41,-6.,-0.74));
#20349=CARTESIAN_POINT('',(-45.17,-6.,-0.5));
#20350=CARTESIAN_POINT('',(-45.65,-6.,-0.98));
#20351=CARTESIAN_POINT('Origin',(0.,-5.75,0.));
#20352=CARTESIAN_POINT('',(-19.9759916874447,-5.5,-0.979671426113));
#20353=CARTESIAN_POINT('Origin',(0.,-5.5,0.));
#20354=CARTESIAN_POINT('Ctrl Pts',(-20.2359894539709,-5.74912062451896,
-0.729120624518967));
#20355=CARTESIAN_POINT('Ctrl Pts',(-20.1051859468429,-5.62294071733704,
-0.855171413339538));
#20356=CARTESIAN_POINT('Ctrl Pts',(-19.9759916874447,-5.5,-0.979671426112999));
#20357=CARTESIAN_POINT('Origin',(-45.65,-6.,-6.));
#20358=CARTESIAN_POINT('',(-45.65,-6.,-4.));
#20359=CARTESIAN_POINT('Origin',(0.,5.75,0.));
#20360=CARTESIAN_POINT('',(-19.9759916874447,5.5,-0.979671426113));
#20361=CARTESIAN_POINT('Ctrl Pts',(-19.9759916874447,5.5,-0.979671426113));
#20362=CARTESIAN_POINT('Ctrl Pts',(-20.1051859468429,5.62294071733699,-0.85517141333958));
#20363=CARTESIAN_POINT('Ctrl Pts',(-20.2359894539709,5.74912062451896,-0.729120624518964));
#20364=CARTESIAN_POINT('Origin',(0.,5.5,0.));
#20365=CARTESIAN_POINT('Origin',(0.,-6.,0.));
#20366=CARTESIAN_POINT('',(-19.9759916874447,-6.,-0.979671426113));
#20367=CARTESIAN_POINT('',(4.91078361144855,-3.48,-19.3877333466687));
#20368=CARTESIAN_POINT('',(4.91078361144856,3.48,-19.3877333466687));
#20369=CARTESIAN_POINT('',(4.91078361144855,-6.,-19.3877333466687));
#20370=CARTESIAN_POINT('',(-4.91078361144855,-3.48,-19.3877333466687));
#20371=CARTESIAN_POINT('Origin',(0.,-3.48,0.));
#20372=CARTESIAN_POINT('',(-4.91078361144855,3.48,-19.3877333466687));
#20373=CARTESIAN_POINT('',(-4.91078361144855,-6.,-19.3877333466687));
#20374=CARTESIAN_POINT('Origin',(0.,3.48,0.));
#20375=CARTESIAN_POINT('Origin',(-20.2248703552884,-6.,-0.7398357130565));
#20376=CARTESIAN_POINT('',(-20.4737490231322,-6.,-0.5));
#20377=CARTESIAN_POINT('Origin',(-4.91744041005317,-6.,-19.4438666733343));
#20378=CARTESIAN_POINT('',(-4.92409720865779,-3.36789585050059,-19.5));
#20379=CARTESIAN_POINT('Ctrl Pts',(-4.91078361144855,-3.48,-19.3877333466687));
#20380=CARTESIAN_POINT('Ctrl Pts',(-4.91522154689806,-3.44263314413296,
-19.4251561523001));
#20381=CARTESIAN_POINT('Ctrl Pts',(-4.91965948264541,-3.40526449477787,
-19.4625789604431));
#20382=CARTESIAN_POINT('Ctrl Pts',(-4.92409720865779,-3.36789585050059,
-19.5));
#20383=CARTESIAN_POINT('',(-4.92409720865779,3.36789585050059,-19.5));
#20384=CARTESIAN_POINT('',(-4.92409720865779,-6.,-19.5));
#20385=CARTESIAN_POINT('Ctrl Pts',(-4.92409720865779,3.36789585050059,-19.5));
#20386=CARTESIAN_POINT('Ctrl Pts',(-4.91965948264339,3.40526449479487,-19.4625789604261));
#20387=CARTESIAN_POINT('Ctrl Pts',(-4.91522154689707,3.44263314414129,-19.4251561522918));
#20388=CARTESIAN_POINT('Ctrl Pts',(-4.91078361144855,3.48,-19.3877333466687));
#20389=CARTESIAN_POINT('Origin',(4.91744041005317,-6.,-19.4438666733343));
#20390=CARTESIAN_POINT('',(4.92409720865779,3.36789585050059,-19.5));
#20391=CARTESIAN_POINT('Ctrl Pts',(4.91078361144855,3.48,-19.3877333466687));
#20392=CARTESIAN_POINT('Ctrl Pts',(4.9152215468944,3.44263314416375,-19.4251561522693));
#20393=CARTESIAN_POINT('Ctrl Pts',(4.91965948263797,3.4052644948405,-19.4625789603804));
#20394=CARTESIAN_POINT('Ctrl Pts',(4.92409720865779,3.36789585050059,-19.5));
#20395=CARTESIAN_POINT('',(4.92409720865779,-3.36789585050059,-19.5));
#20396=CARTESIAN_POINT('',(4.92409720865779,-6.,-19.5));
#20397=CARTESIAN_POINT('Ctrl Pts',(4.92409720865779,-3.36789585050059,-19.5));
#20398=CARTESIAN_POINT('Ctrl Pts',(4.91965948264544,-3.40526449477763,-19.4625789604433));
#20399=CARTESIAN_POINT('Ctrl Pts',(4.91522154689809,-3.44263314413272,-19.4251561523004));
#20400=CARTESIAN_POINT('Ctrl Pts',(4.91078361144855,-3.48,-19.3877333466687));
#20401=CARTESIAN_POINT('Origin',(0.,3.24,0.));
#20402=CARTESIAN_POINT('',(-6.25942489371028,3.,-19.5));
#20403=CARTESIAN_POINT('',(6.25942489371028,3.,-19.5));
#20404=CARTESIAN_POINT('Origin',(0.,3.,0.));
#20405=CARTESIAN_POINT('Ctrl Pts',(6.25942489371028,3.00000000000001,-19.5));
#20406=CARTESIAN_POINT('Ctrl Pts',(5.58570985570301,3.20591155664892,-19.5));
#20407=CARTESIAN_POINT('Ctrl Pts',(4.92409720865779,3.36789585050059,-19.5));
#20408=CARTESIAN_POINT('Ctrl Pts',(-4.92409720865779,3.3678958505006,-19.5));
#20409=CARTESIAN_POINT('Ctrl Pts',(-5.58570985570301,3.20591155664892,-19.5));
#20410=CARTESIAN_POINT('Ctrl Pts',(-6.25942489371029,3.,-19.5));
#20411=CARTESIAN_POINT('Origin',(0.,-3.24,0.));
#20412=CARTESIAN_POINT('',(6.25942489371028,-3.,-19.5));
#20413=CARTESIAN_POINT('Ctrl Pts',(4.92409720865779,-3.36789585050059,-19.5));
#20414=CARTESIAN_POINT('Ctrl Pts',(5.58570985570301,-3.20591155664891,-19.5));
#20415=CARTESIAN_POINT('Ctrl Pts',(6.25942489371028,-3.,-19.5));
#20416=CARTESIAN_POINT('',(-6.25942489371028,-3.,-19.5));
#20417=CARTESIAN_POINT('Origin',(0.,-3.,0.));
#20418=CARTESIAN_POINT('Ctrl Pts',(-6.25942489371028,-3.,-19.5));
#20419=CARTESIAN_POINT('Ctrl Pts',(-5.58570985570301,-3.20591155664891,
-19.5));
#20420=CARTESIAN_POINT('Ctrl Pts',(-4.92409720865778,-3.36789585050059,
-19.5));
#20421=CARTESIAN_POINT('Origin',(0.,-3.,-25.25));
#20422=CARTESIAN_POINT('',(11.,-3.,-19.5));
#20423=CARTESIAN_POINT('',(11.,-3.,-19.5));
#20424=CARTESIAN_POINT('',(11.,-3.,-27.3939847411799));
#20425=CARTESIAN_POINT('',(11.,-3.,-31.));
#20426=CARTESIAN_POINT('',(-11.,-3.,-27.3939847411799));
#20427=CARTESIAN_POINT('Origin',(0.,-3.,0.));
#20428=CARTESIAN_POINT('',(-11.,-3.,-19.5));
#20429=CARTESIAN_POINT('',(-11.,-3.,-19.5));
#20430=CARTESIAN_POINT('',(11.,-3.,-19.5));
#20431=CARTESIAN_POINT('Origin',(-11.,-3.,-19.5));
#20432=CARTESIAN_POINT('',(11.,3.,-19.5));
#20433=CARTESIAN_POINT('',(11.,3.,-19.5));
#20434=CARTESIAN_POINT('',(11.,-3.,-19.5));
#20435=CARTESIAN_POINT('Origin',(-11.2225734265705,-6.,-27.5807880133765));
#20436=CARTESIAN_POINT('',(-11.445146853141,-3.48,-27.7310045528473));
#20437=CARTESIAN_POINT('',(-11.445146853141,3.48,-27.7310045528473));
#20438=CARTESIAN_POINT('',(-11.445146853141,-6.,-27.7310045528473));
#20439=CARTESIAN_POINT('',(-11.,3.03395491952051,-27.4305714739057));
#20440=CARTESIAN_POINT('Ctrl Pts',(-11.445146853141,3.48,-27.7310045528473));
#20441=CARTESIAN_POINT('Ctrl Pts',(-11.2969785213058,3.33103640993591,-27.6310045914395));
#20442=CARTESIAN_POINT('Ctrl Pts',(-11.14857662724,3.1823261888354,-27.5308469970628));
#20443=CARTESIAN_POINT('Ctrl Pts',(-11.,3.03395491952051,-27.4305714739057));
#20444=CARTESIAN_POINT('',(-11.,-3.03395491952051,-27.4305714739057));
#20445=CARTESIAN_POINT('',(-11.,-6.,-27.4305714739057));
#20446=CARTESIAN_POINT('Ctrl Pts',(-11.,-3.03395491952051,-27.4305714739057));
#20447=CARTESIAN_POINT('Ctrl Pts',(-11.14857662724,-3.18232618883539,-27.5308469970628));
#20448=CARTESIAN_POINT('Ctrl Pts',(-11.2969785213057,-3.33103640993588,
-27.6310045914395));
#20449=CARTESIAN_POINT('Ctrl Pts',(-11.445146853141,-3.48,-27.7310045528473));
#20450=CARTESIAN_POINT('Origin',(11.2225734265705,-6.,-27.5807880133765));
#20451=CARTESIAN_POINT('',(11.445146853141,3.48,-27.7310045528473));
#20452=CARTESIAN_POINT('',(11.445146853141,-3.48,-27.7310045528473));
#20453=CARTESIAN_POINT('',(11.445146853141,-6.,-27.7310045528473));
#20454=CARTESIAN_POINT('',(11.,-3.03395491952051,-27.4305714739057));
#20455=CARTESIAN_POINT('Ctrl Pts',(11.445146853141,-3.48,-27.7310045528473));
#20456=CARTESIAN_POINT('Ctrl Pts',(11.2969785213068,-3.33103640993696,-27.6310045914402));
#20457=CARTESIAN_POINT('Ctrl Pts',(11.1485766272405,-3.1823261888359,-27.5308469970632));
#20458=CARTESIAN_POINT('Ctrl Pts',(11.,-3.03395491952051,-27.4305714739057));
#20459=CARTESIAN_POINT('',(11.,3.03395491952051,-27.4305714739057));
#20460=CARTESIAN_POINT('',(11.,-6.,-27.4305714739057));
#20461=CARTESIAN_POINT('Ctrl Pts',(11.,3.03395491952051,-27.4305714739057));
#20462=CARTESIAN_POINT('Ctrl Pts',(11.1485766272405,3.18232618883592,-27.5308469970632));
#20463=CARTESIAN_POINT('Ctrl Pts',(11.2969785213068,3.33103640993699,-27.6310045914402));
#20464=CARTESIAN_POINT('Ctrl Pts',(11.445146853141,3.48,-27.7310045528473));
#20465=CARTESIAN_POINT('Origin',(0.,-3.24,0.));
#20466=CARTESIAN_POINT('Ctrl Pts',(11.,-3.,-27.39398474118));
#20467=CARTESIAN_POINT('Ctrl Pts',(11.,-3.01696612998714,-27.4122675927604));
#20468=CARTESIAN_POINT('Ctrl Pts',(11.,-3.0339549195205,-27.4305714739057));
#20469=CARTESIAN_POINT('Origin',(0.,-3.48,0.));
#20470=CARTESIAN_POINT('Ctrl Pts',(-11.,-3.0339549195205,-27.4305714739057));
#20471=CARTESIAN_POINT('Ctrl Pts',(-11.,-3.01696612998714,-27.4122675927604));
#20472=CARTESIAN_POINT('Ctrl Pts',(-11.,-2.99999999999999,-27.3939847411799));
#20473=CARTESIAN_POINT('Origin',(0.,3.24,0.));
#20474=CARTESIAN_POINT('Origin',(0.,3.48,0.));
#20475=CARTESIAN_POINT('',(11.,3.,-27.3939847411799));
#20476=CARTESIAN_POINT('Ctrl Pts',(11.,3.03395491952051,-27.4305714739057));
#20477=CARTESIAN_POINT('Ctrl Pts',(11.,3.01696612998715,-27.4122675927604));
#20478=CARTESIAN_POINT('Ctrl Pts',(11.,3.,-27.3939847411799));
#20479=CARTESIAN_POINT('',(-11.,3.,-27.3939847411799));
#20480=CARTESIAN_POINT('Origin',(0.,3.,0.));
#20481=CARTESIAN_POINT('Ctrl Pts',(-11.,3.,-27.3939847411799));
#20482=CARTESIAN_POINT('Ctrl Pts',(-11.,3.01696612998714,-27.4122675927604));
#20483=CARTESIAN_POINT('Ctrl Pts',(-11.,3.03395491952051,-27.4305714739057));
#20484=CARTESIAN_POINT('Origin',(0.,3.,-25.25));
#20485=CARTESIAN_POINT('',(-11.,3.,-19.5));
#20486=CARTESIAN_POINT('',(11.,3.,-19.5));
#20487=CARTESIAN_POINT('',(-11.,3.,-19.5));
#20488=CARTESIAN_POINT('',(11.,3.,-31.));
#20489=CARTESIAN_POINT('Origin',(11.,-3.,-19.5));
#20490=CARTESIAN_POINT('Origin',(0.,-6.,0.));
#20491=CARTESIAN_POINT('Origin',(0.,5.5,0.));
#20492=CARTESIAN_POINT('Origin',(0.,-5.5,0.));
#20493=CARTESIAN_POINT('Origin',(0.,5.75,0.));
#20494=CARTESIAN_POINT('Origin',(29.9958330439413,-6.,-0.5));
#20495=CARTESIAN_POINT('',(-41.75,-2.75545529808155E-16,-0.5));
#20496=CARTESIAN_POINT('Origin',(-39.5,0.,-0.5));
#20497=CARTESIAN_POINT('Origin',(0.,-5.75,0.));
#20498=CARTESIAN_POINT('Origin',(-11.,-3.,-31.));
#20499=CARTESIAN_POINT('',(-11.,-3.,-19.5));
#20500=CARTESIAN_POINT('Origin',(-11.,-3.,-19.5));
#20501=CARTESIAN_POINT('Origin',(39.5,0.,-0.5));
#20502=CARTESIAN_POINT('',(37.25,2.75545529808154E-16,-0.5));
#20503=CARTESIAN_POINT('Origin',(-39.5,0.,-0.5));
#20504=CARTESIAN_POINT('',(-41.75,-2.75545529808155E-16,-6.));
#20505=CARTESIAN_POINT('',(-41.75,2.75545529808155E-16,-0.5));
#20506=CARTESIAN_POINT('Origin',(-39.5,0.,-6.));
#20507=CARTESIAN_POINT('Origin',(-34.4,0.,-33.));
#20508=CARTESIAN_POINT('',(-34.4,-2.63299061816681E-16,-30.85));
#20509=CARTESIAN_POINT('Origin',(-34.4,0.,-33.));
#20510=CARTESIAN_POINT('',(-34.4,-2.63299061816681E-16,-30.85));
#20511=CARTESIAN_POINT('Origin',(34.4,0.,-33.));
#20512=CARTESIAN_POINT('',(34.4,2.63299061816681E-16,-30.85));
#20513=CARTESIAN_POINT('Origin',(17.2,-2.,-34.5));
#20514=CARTESIAN_POINT('',(17.2,-2.,-38.5));
#20515=CARTESIAN_POINT('Origin',(17.2,2.,-34.5));
#20516=CARTESIAN_POINT('',(17.2,2.,-38.5));
#20517=CARTESIAN_POINT('Origin',(-43.65,-6.,-4.));
#20518=CARTESIAN_POINT('',(-43.65,-6.,-6.));
#20519=CARTESIAN_POINT('Origin',(-34.4,-6.,-6.));
#20520=CARTESIAN_POINT('',(-34.4,-6.,-6.));
#20521=CARTESIAN_POINT('Origin',(34.4,-6.,-38.5));
#20522=CARTESIAN_POINT('Origin',(-34.4,-6.,-38.5));
#37154=UNCERTAINTY_MEASURE_WITH_UNIT(LENGTH_MEASURE(0.01),#37182,
'DISTANCE_ACCURACY_VALUE',
'Maximum model space distance between geometric entities at asserted c
onnectivities');
#37166=UNCERTAINTY_MEASURE_WITH_UNIT(LENGTH_MEASURE(0.01),#37182,
'DISTANCE_ACCURACY_VALUE',
'Maximum model space distance between geometric entities at asserted c
onnectivities');
#37169=(
GEOMETRIC_REPRESENTATION_CONTEXT(3)
GLOBAL_UNCERTAINTY_ASSIGNED_CONTEXT((#37154))
GLOBAL_UNIT_ASSIGNED_CONTEXT((#37182,#37184,#37185))
REPRESENTATION_CONTEXT('','3D')
);
#37181=(
GEOMETRIC_REPRESENTATION_CONTEXT(3)
GLOBAL_UNCERTAINTY_ASSIGNED_CONTEXT((#37166))
GLOBAL_UNIT_ASSIGNED_CONTEXT((#37182,#37184,#37185))
REPRESENTATION_CONTEXT('','3D')
);
#37182=(
LENGTH_UNIT()
NAMED_UNIT(*)
SI_UNIT(.MILLI.,.METRE.)
);
#37184=(
NAMED_UNIT(*)
PLANE_ANGLE_UNIT()
SI_UNIT($,.RADIAN.)
);
#37185=(
NAMED_UNIT(*)
SI_UNIT($,.STERADIAN.)
SOLID_ANGLE_UNIT()
);
#37188=SHAPE_DEFINITION_REPRESENTATION(#37202,#37239);
#37202=PRODUCT_DEFINITION_SHAPE('',$,#37254);
#37239=SHAPE_REPRESENTATION('',(#14997),#37169);
#37251=PRODUCT_DEFINITION_CONTEXT('part definition',#37295,'design');
#37254=PRODUCT_DEFINITION('2026-10-20-13-23-47-919',
'02_Clamp_Lower_Half_with_Legs_PLA',#37268,#37251);
#37268=PRODUCT_DEFINITION_FORMATION('',$,#37299);
#37295=APPLICATION_CONTEXT(
'Core Data for Automotive Mechanical Design Process');
#37296=PRODUCT_CONTEXT('part definition',#37295,'mechanical');
#37299=PRODUCT('2026-10-20-13-23-47-919',
'02_Clamp_Lower_Half_with_Legs_PLA',$,(#37296));
#37381=COLOUR_RGB('Off White',0.89,0.88,0.83);
#37382=FILL_AREA_STYLE_COLOUR('',#37381);
#37383=FILL_AREA_STYLE('',(#37382));
#37384=SURFACE_STYLE_FILL_AREA(#37383);
#37385=SURFACE_SIDE_STYLE('',(#37384));
#37386=SURFACE_STYLE_USAGE(.BOTH.,#37385);
#37387=PRESENTATION_STYLE_ASSIGNMENT((#37386));
ENDSEC;
END-ISO-10303-21;
